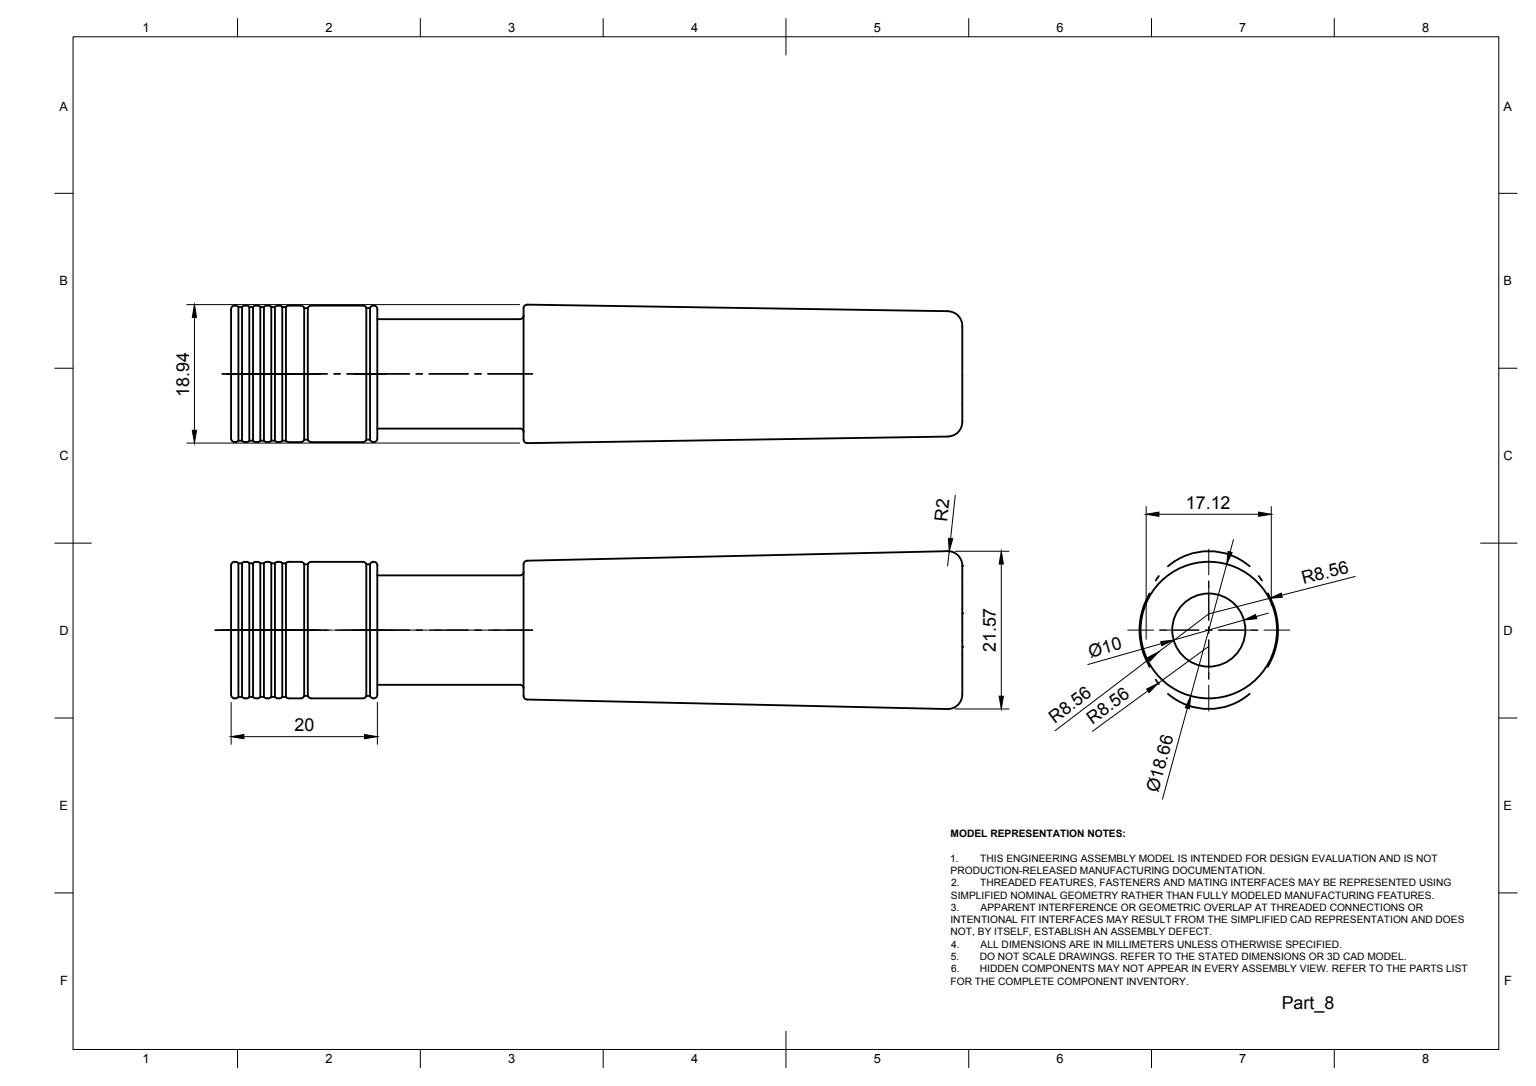
ISO-10303-21;
HEADER;
/* Generated by software containing ST-Developer
 * from STEP Tools, Inc. (www.steptools.com) 
 */

FILE_DESCRIPTION(
/* description */ ('STEP AP242 Edition 2'),
/* implementation_level */ '2;1');

FILE_NAME(
/* name */ 'Part_8.step',
/* time_stamp */ '2026-10-06T10:11:12-07:00',
/* author */ (''),
/* organization */ (''),
/* preprocessor_version */ 'ST-DEVELOPER v20.2',
/* originating_system */ 'Autodesk Translation Framework v15.15.0.0',
/* authorisation */ '');

FILE_SCHEMA (('AUTOMOTIVE_DESIGN { 1 0 10303 214 3 1 1 }'));
ENDSEC;

DATA;
#10=MECHANICAL_DESIGN_GEOMETRIC_PRESENTATION_REPRESENTATION('',(#1772,#1773,#1774,#1775,#1776,#1777,#1778,#1779,#1780,#1781,#1782,#1783,#1784),#54580);
#171=TOROIDAL_SURFACE('',#18476,0.00656151574957875,0.00199999992126171);
#172=TOROIDAL_SURFACE('',#18477,0.0065615157495791,0.00199999992126177);
#173=TOROIDAL_SURFACE('',#18479,0.0079756477610481,0.0005);
#174=TOROIDAL_SURFACE('',#18481,0.0045,0.0005);
#175=TOROIDAL_SURFACE('',#18483,0.0055,0.0005);
#176=TOROIDAL_SURFACE('',#18485,0.00882888901198444,0.0005);
#177=TOROIDAL_SURFACE('',#18487,0.00882888901198444,0.0005);
#178=TOROIDAL_SURFACE('',#18489,0.00882888901198444,0.0005);
#179=TOROIDAL_SURFACE('',#18491,0.00882888901198444,0.0005);
#180=TOROIDAL_SURFACE('',#18493,0.00882888901198444,0.0005);
#181=TOROIDAL_SURFACE('',#18495,0.00882888901198444,0.0005);
#182=TOROIDAL_SURFACE('',#18497,0.00882888901198444,0.0005);
#183=TOROIDAL_SURFACE('',#18499,0.00882888901198444,0.0005);
#184=TOROIDAL_SURFACE('',#18501,0.00882888901198444,0.0005);
#185=TOROIDAL_SURFACE('',#18503,0.00882888901198444,0.0005);
#186=TOROIDAL_SURFACE('',#18505,0.00882888901198444,0.0005);
#187=TOROIDAL_SURFACE('',#18507,0.00882888901198444,0.0005);
#188=TOROIDAL_SURFACE('',#18509,0.00882888901198444,0.0005);
#189=TOROIDAL_SURFACE('',#18511,0.00882888901198444,0.0005);
#190=TOROIDAL_SURFACE('',#18513,0.00882888901198444,0.0005);
#191=TOROIDAL_SURFACE('',#18515,0.00882888901198444,0.0005);
#323=B_SPLINE_SURFACE_WITH_KNOTS('',3,1,((#25149,#25150),(#25151,#25152),
(#25153,#25154),(#25155,#25156),(#25157,#25158),(#25159,#25160),(#25161,
#25162),(#25163,#25164),(#25165,#25166),(#25167,#25168),(#25169,#25170),
(#25171,#25172),(#25173,#25174),(#25175,#25176),(#25177,#25178),(#25179,
#25180),(#25181,#25182),(#25183,#25184),(#25185,#25186),(#25187,#25188),
(#25189,#25190),(#25191,#25192),(#25193,#25194),(#25195,#25196),(#25197,
#25198),(#25199,#25200),(#25201,#25202),(#25203,#25204),(#25205,#25206),
(#25207,#25208)),.UNSPECIFIED.,.T.,.F.,.F.,(4,1,1,1,1,1,1,1,2,1,1,1,2,1,
1,1,1,1,1,1,2,1,1,1,4),(2,2),(-1.,-0.94727121518274,-0.894542430365479,
-0.841813645548218,-0.789084860730959,-0.736356075913698,-0.683627291096437,
-0.630898506279177,-0.578169721461916,-0.558627291096437,-0.539084860730958,
-0.519542430365479,-0.5,-0.447271215182739,-0.394542430365479,-0.341813645548219,
-0.289084860730958,-0.236356075913698,-0.183627291096437,-0.130898506279177,
-0.078169721461917,-0.0586272910964371,-0.039084860730958,-0.019542430365479,
0.),(0.0270596808612465,0.997611167870436),.UNSPECIFIED.);
#324=B_SPLINE_SURFACE_WITH_KNOTS('',3,1,((#25444,#25445),(#25446,#25447),
(#25448,#25449),(#25450,#25451),(#25452,#25453),(#25454,#25455),(#25456,
#25457),(#25458,#25459),(#25460,#25461),(#25462,#25463),(#25464,#25465),
(#25466,#25467),(#25468,#25469),(#25470,#25471),(#25472,#25473),(#25474,
#25475),(#25476,#25477),(#25478,#25479),(#25480,#25481),(#25482,#25483),
(#25484,#25485),(#25486,#25487),(#25488,#25489),(#25490,#25491),(#25492,
#25493),(#25494,#25495),(#25496,#25497),(#25498,#25499),(#25500,#25501),
(#25502,#25503)),.UNSPECIFIED.,.T.,.F.,.F.,(4,1,1,1,1,1,1,1,2,1,1,1,2,1,
1,1,1,1,1,1,2,1,1,1,4),(2,2),(0.,0.0527287848172604,0.105457569634521,0.158186354451782,
0.210915139269041,0.263643924086302,0.316372708903563,0.369101493720823,
0.421830278538084,0.441372708903563,0.460915139269042,0.480457569634521,
0.5,0.552728784817261,0.605457569634521,0.658186354451781,0.710915139269042,
0.763643924086302,0.816372708903563,0.869101493720823,0.921830278538083,
0.941372708903563,0.960915139269042,0.980457569634521,1.),(0.0270596808612465,
0.997611167870436),.UNSPECIFIED.);
#343=B_SPLINE_CURVE_WITH_KNOTS('',3,(#24904,#24905,#24906,#24907,#24908,
#24909,#24910,#24911,#24912,#24913,#24914,#24915,#24916,#24917,#24918,#24919,
#24920,#24921,#24922,#24923,#24924,#24925,#24926,#24927,#24928,#24929,#24930,
#24931,#24932,#24933,#24934,#24935,#24936,#24937,#24938,#24939,#24940,#24941,
#24942,#24943,#24944,#24945,#24946,#24947,#24948,#24949,#24950,#24951,#24952,
#24953,#24954,#24955,#24956,#24957,#24958,#24959,#24960,#24961,#24962,#24963,
#24964,#24965,#24966,#24967,#24968,#24969,#24970,#24971,#24972,#24973,#24974,
#24975,#24976,#24977,#24978,#24979,#24980,#24981,#24982,#24983,#24984,#24985,
#24986,#24987,#24988,#24989,#24990,#24991,#24992,#24993,#24994,#24995,#24996,
#24997,#24998,#24999,#25000,#25001,#25002,#25003,#25004,#25005,#25006,#25007,
#25008,#25009,#25010,#25011,#25012,#25013,#25014,#25015,#25016,#25017,#25018,
#25019,#25020,#25021,#25022,#25023,#25024,#25025,#25026,#25027,#25028,#25029,
#25030,#25031,#25032,#25033,#25034,#25035,#25036,#25037,#25038,#25039,#25040,
#25041,#25042,#25043,#25044,#25045),.UNSPECIFIED.,.F.,.F.,(4,3,3,3,3,3,
3,3,3,3,3,3,3,3,3,3,3,3,3,3,3,3,3,3,3,3,3,3,3,3,3,3,3,3,3,3,3,3,3,3,3,3,
3,3,3,3,3,4),(1.65573441350565E-7,0.00176667375437257,0.00259221926243185,
0.00265001063155886,0.00353334750874515,0.00441668438593144,0.00612523623771844,
0.0070666950174903,0.00965970053988215,0.0106000425262354,0.0114833794034217,
0.0131911273471506,0.0141333900349806,0.0150167269121669,0.0167215202745876,
0.0176667375437257,0.018550074420912,0.0202567299474385,0.0212000850524709,
0.0220834219296572,0.0237972002706092,0.024733432561216,0.0265001063155886,
0.0273265094643739,0.0273834431927749,0.0282667800699612,0.0291501169471475,
0.0308585741103488,0.0318001275787063,0.0326834644558926,0.0343965954050026,
0.0353334750874515,0.0379347075752174,0.0388668225961966,0.0397501594733829,
0.0414708448549527,0.0424001701049418,0.0432835069821281,0.0450045160112871,
0.0459335176136869,0.0468168544908732,0.0485354593167441,0.0494668651224321,
0.0503502019996184,0.052066506161832,0.0530002126311772,0.0538835495083635,
0.0555994356637866),.UNSPECIFIED.);
#344=B_SPLINE_CURVE_WITH_KNOTS('',3,(#25051,#25052,#25053,#25054,#25055,
#25056,#25057,#25058,#25059,#25060,#25061,#25062,#25063,#25064,#25065,#25066,
#25067,#25068,#25069,#25070,#25071,#25072,#25073,#25074,#25075,#25076,#25077,
#25078,#25079,#25080,#25081,#25082,#25083,#25084,#25085,#25086,#25087,#25088,
#25089,#25090,#25091,#25092,#25093,#25094,#25095,#25096,#25097,#25098,#25099,
#25100,#25101,#25102,#25103,#25104,#25105,#25106,#25107,#25108,#25109,#25110,
#25111,#25112,#25113,#25114,#25115,#25116,#25117),.UNSPECIFIED.,.F.,.F.,
(4,3,3,3,3,3,3,3,3,3,3,3,3,3,3,3,3,3,3,3,3,3,4),(0.0193063570369876,0.0197413378854143,
0.0225007291837996,0.0234952979646733,0.0262508507144329,0.0272500609140882,
0.0300009722450662,0.0309993547899246,0.0337510937756994,0.0347455027219703,
0.0375012153063327,0.0385033658381765,0.041251336836966,0.0422556599874251,
0.0450014583675992,0.0460030914440076,0.0487515798982325,0.0497511536421023,
0.0525017014288658,0.053501189887995,0.0562518229594991,0.057250590934481,
0.0600019444901323),.UNSPECIFIED.);
#345=B_SPLINE_CURVE_WITH_KNOTS('',3,(#25118,#25119,#25120,#25121,#25122,
#25123,#25124,#25125,#25126,#25127,#25128,#25129,#25130,#25131,#25132,#25133,
#25134,#25135,#25136,#25137,#25138,#25139,#25140,#25141,#25142,#25143,#25144,
#25145,#25146,#25147,#25148),.UNSPECIFIED.,.F.,.F.,(4,3,3,3,3,3,3,3,3,3,
4),(0.000991839717425502,0.00375012153063327,0.00474188317058086,0.00750024306126654,
0.00848950942012792,0.0112503645918998,0.0122372989824959,0.0150004861225331,
0.0159882081557064,0.0187506076531663,0.0193063570369876),.UNSPECIFIED.);
#346=B_SPLINE_CURVE_WITH_KNOTS('',1,(#25210,#25211),.UNSPECIFIED.,.F.,.F.,
(2,2),(-0.991582441935872,-0.0329929514257554),.UNSPECIFIED.);
#347=B_SPLINE_CURVE_WITH_KNOTS('',1,(#25213,#25214),.UNSPECIFIED.,.F.,.F.,
(2,2),(-0.991765438998876,-0.0337011078849239),.UNSPECIFIED.);
#348=B_SPLINE_CURVE_WITH_KNOTS('',3,(#25216,#25217,#25218,#25219,#25220,
#25221,#25222,#25223),.UNSPECIFIED.,.F.,.F.,(4,1,1,1,1,4),(0.,0.0625,0.125,
0.15625,0.1875,0.214595707386903),.UNSPECIFIED.);
#349=B_SPLINE_CURVE_WITH_KNOTS('',3,(#25225,#25226,#25227,#25228,#25229,
#25230,#25231,#25232,#25233,#25234,#25235,#25236,#25237,#25238,#25239,#25240,
#25241,#25242,#25243),.UNSPECIFIED.,.F.,.F.,(4,3,3,3,3,3,4),(1.18815451677939E-5,
0.00305752378009468,0.257254477967242,0.499999999995986,0.742745522020828,
0.996942476194294,0.99998811883621),.UNSPECIFIED.);
#350=B_SPLINE_CURVE_WITH_KNOTS('',3,(#25245,#25246,#25247,#25248,#25249,
#25250,#25251,#25252,#25253,#25254,#25255,#25256,#25257,#25258,#25259,#25260,
#25261,#25262,#25263,#25264,#25265,#25266,#25267,#25268,#25269,#25270,#25271,
#25272,#25273,#25274,#25275,#25276,#25277,#25278,#25279),.UNSPECIFIED.,
 .F.,.F.,(4,1,1,1,1,1,1,1,1,1,1,1,1,1,1,1,1,1,1,1,1,1,1,1,1,1,1,1,1,1,1,
1,4),(0.,0.0625,0.125,0.15625,0.1875,0.21875,0.234375,0.2421875,0.25,0.2578125,
0.265625,0.28125,0.3125,0.34375,0.375,0.4375,0.5,0.5625,0.625,0.65625,0.6875,
0.71875,0.734375,0.7421875,0.75,0.7578125,0.765625,0.78125,0.8125,0.84375,
0.875,0.9375,1.),.UNSPECIFIED.);
#351=B_SPLINE_CURVE_WITH_KNOTS('',3,(#25280,#25281,#25282,#25283,#25284,
#25285,#25286,#25287,#25288,#25289,#25290,#25291,#25292,#25293,#25294,#25295),
 .UNSPECIFIED.,.F.,.F.,(4,3,3,3,3,4),(0.00305752354988625,0.25725447786239,
0.499999999961484,0.742745522020858,0.996942476194068,0.999988118836217),
 .UNSPECIFIED.);
#352=B_SPLINE_CURVE_WITH_KNOTS('',3,(#25505,#25506,#25507,#25508),
 .UNSPECIFIED.,.F.,.F.,(4,4),(1.18815450203416E-5,0.00305752354988625),
 .UNSPECIFIED.);
#353=B_SPLINE_CURVE_WITH_KNOTS('',3,(#25509,#25510,#25511,#25512,#25513,
#25514,#25515,#25516,#25517,#25518,#25519,#25520,#25521,#25522,#25523,#25524,
#25525,#25526,#25527,#25528,#25529,#25530,#25531,#25532,#25533,#25534,#25535,
#25536,#25537,#25538,#25539),.UNSPECIFIED.,.F.,.F.,(4,1,1,1,1,1,1,1,1,1,
1,1,1,1,1,1,1,1,1,1,1,1,1,1,1,1,1,1,4),(0.214595707386903,0.21875,0.234375,
0.2421875,0.25,0.2578125,0.265625,0.28125,0.3125,0.34375,0.375,0.4375,0.5,
0.5625,0.625,0.65625,0.6875,0.71875,0.734375,0.7421875,0.75,0.7578125,0.765625,
0.78125,0.8125,0.84375,0.875,0.9375,1.),.UNSPECIFIED.);
#354=B_SPLINE_CURVE_WITH_KNOTS('',3,(#25540,#25541,#25542,#25543),
 .UNSPECIFIED.,.F.,.F.,(4,4),(0.,0.000991839717425502),.UNSPECIFIED.);
#355=B_SPLINE_CURVE_WITH_KNOTS('',3,(#25546,#25547,#25548,#25549),
 .UNSPECIFIED.,.F.,.F.,(4,4),(0.,1.65573441350565E-7),.UNSPECIFIED.);
#356=B_SPLINE_CURVE_WITH_KNOTS('',3,(#25550,#25551,#25552,#25553),
 .UNSPECIFIED.,.F.,.F.,(4,4),(0.0555994356637866,0.0565335601399224),
 .UNSPECIFIED.);
#357=B_SPLINE_CURVE_WITH_KNOTS('',3,(#25562,#25563,#25564,#25565,#25566,
#25567,#25568,#25569,#25570,#25571,#25572,#25573,#25574,#25575,#25576,#25577,
#25578,#25579,#25580,#25581,#25582,#25583,#25584,#25585,#25586),
 .UNSPECIFIED.,.F.,.F.,(4,3,3,3,3,3,3,3,4),(0.,0.144356336537315,0.25,0.395552475785214,
0.5,0.64383331940147,0.75,0.898848831223356,1.),.UNSPECIFIED.);
#358=B_SPLINE_CURVE_WITH_KNOTS('',3,(#25588,#25589,#25590,#25591,#25592,
#25593,#25594,#25595,#25596,#25597,#25598,#25599,#25600,#25601,#25602,#25603,
#25604,#25605,#25606,#25607,#25608,#25609,#25610,#25611,#25612,#25613,#25614,
#25615,#25616,#25617,#25618,#25619,#25620,#25621,#25622,#25623,#25624),
 .UNSPECIFIED.,.F.,.F.,(4,3,3,3,3,3,3,3,3,3,3,3,4),(0.,0.125,0.1875,0.25,
0.3125,0.375,0.5,0.625,0.6875,0.75,0.8125,0.875,1.),.UNSPECIFIED.);
#359=B_SPLINE_CURVE_WITH_KNOTS('',3,(#25626,#25627,#25628,#25629,#25630,
#25631,#25632,#25633,#25634,#25635,#25636,#25637,#25638,#25639,#25640,#25641,
#25642,#25643,#25644,#25645,#25646,#25647,#25648,#25649,#25650),
 .UNSPECIFIED.,.F.,.F.,(4,3,3,3,3,3,3,3,4),(0.,0.144356336542805,0.25,0.395552475791052,
0.5,0.643833319408362,0.75,0.898848831228882,1.),.UNSPECIFIED.);
#360=B_SPLINE_CURVE_WITH_KNOTS('',3,(#25651,#25652,#25653,#25654,#25655,
#25656,#25657,#25658,#25659,#25660,#25661,#25662,#25663,#25664,#25665,#25666,
#25667,#25668,#25669,#25670,#25671,#25672,#25673,#25674,#25675,#25676,#25677,
#25678,#25679,#25680,#25681,#25682,#25683,#25684,#25685,#25686,#25687),
 .UNSPECIFIED.,.F.,.F.,(4,3,3,3,3,3,3,3,3,3,3,3,4),(0.,0.125,0.1875,0.25,
0.3125,0.375,0.5,0.625,0.6875,0.75,0.8125,0.875,1.),.UNSPECIFIED.);
#361=B_SPLINE_CURVE_WITH_KNOTS('',3,(#25689,#25690,#25691,#25692,#25693,
#25694,#25695,#25696,#25697,#25698,#25699,#25700,#25701),.UNSPECIFIED.,
 .F.,.F.,(4,3,3,3,4),(0.,0.393665259181331,0.5,0.894848401742748,0.999999577588646),
 .UNSPECIFIED.);
#362=B_SPLINE_CURVE_WITH_KNOTS('',3,(#25702,#25703,#25704,#25705,#25706,
#25707,#25708,#25709,#25710,#25711,#25712,#25713,#25714),.UNSPECIFIED.,
 .F.,.F.,(4,3,3,3,4),(4.22403003312878E-7,0.394848747914453,0.5,0.89366522956997,
1.),.UNSPECIFIED.);
#363=B_SPLINE_CURVE_WITH_KNOTS('',3,(#25716,#25717,#25718,#25719,#25720,
#25721,#25722,#25723,#25724,#25725,#25726,#25727,#25728),.UNSPECIFIED.,
 .F.,.F.,(4,3,3,3,4),(0.,0.39366525918135,0.5,0.894848401747474,0.999999577588569),
 .UNSPECIFIED.);
#364=B_SPLINE_CURVE_WITH_KNOTS('',3,(#25730,#25731,#25732,#25733,#25734,
#25735,#25736,#25737,#25738,#25739,#25740,#25741,#25742),.UNSPECIFIED.,
 .F.,.F.,(4,3,3,3,4),(4.22402912852314E-7,0.394848747910699,0.5,0.893665229570505,
1.),.UNSPECIFIED.);
#1512=(
BOUNDED_CURVE()
B_SPLINE_CURVE(2,(#24900,#24901,#24902),.UNSPECIFIED.,.F.,.F.)
B_SPLINE_CURVE_WITH_KNOTS((3,3),(-0.99956690722118,-2.51118997643904E-6),
 .UNSPECIFIED.)
CURVE()
GEOMETRIC_REPRESENTATION_ITEM()
RATIONAL_B_SPLINE_CURVE((0.999750853586006,0.71236441613048,0.999998554758888))
REPRESENTATION_ITEM('')
);
#1513=(
BOUNDED_CURVE()
B_SPLINE_CURVE(2,(#25047,#25048,#25049),.UNSPECIFIED.,.F.,.F.)
B_SPLINE_CURVE_WITH_KNOTS((3,3),(-0.999613386882244,0.),.UNSPECIFIED.)
CURVE()
GEOMETRIC_REPRESENTATION_ITEM()
RATIONAL_B_SPLINE_CURVE((0.999776843008427,0.711394956192752,1.))
REPRESENTATION_ITEM('')
);
#1530=(
BOUNDED_SURFACE()
B_SPLINE_SURFACE(3,2,((#24841,#24842,#24843),(#24844,#24845,#24846),(#24847,
#24848,#24849),(#24850,#24851,#24852),(#24853,#24854,#24855),(#24856,#24857,
#24858),(#24859,#24860,#24861),(#24862,#24863,#24864),(#24865,#24866,#24867),
(#24868,#24869,#24870),(#24871,#24872,#24873),(#24874,#24875,#24876),(#24877,
#24878,#24879),(#24880,#24881,#24882),(#24883,#24884,#24885),(#24886,#24887,
#24888),(#24889,#24890,#24891),(#24892,#24893,#24894),(#24895,#24896,#24897)),
 .UNSPECIFIED.,.T.,.F.,.F.)
B_SPLINE_SURFACE_WITH_KNOTS((4,1,1,1,1,1,1,1,1,1,1,1,1,1,1,1,4),(3,3),(-0.056131150341711,
-0.0526229534453541,-0.0491147565489971,-0.0456065596526402,-0.0420983627562833,
-0.0385901658599263,-0.0350819689635694,-0.0315737720672124,-0.0280655751708555,
-0.0245573782744986,-0.0210491813781416,-0.0175409844817847,-0.0140327875854278,
-0.0105245906890708,-0.0070163937927139,-0.003508196896357,0.),(0.,1.),
 .UNSPECIFIED.)
GEOMETRIC_REPRESENTATION_ITEM()
RATIONAL_B_SPLINE_SURFACE(((1.,0.712239066951905,1.),(1.,0.711110760308393,
1.),(1.,0.708331161318748,1.),(1.,0.701023190412799,1.),(1.,0.701644224301599,
1.),(1.,0.70884038203116,1.),(1.,0.712835506198471,1.),(1.,0.715218629500482,
1.),(1.,0.715102433806893,1.),(1.,0.712501311419114,1.),(1.,0.708334487423287,
1.),(1.,0.701010241546403,1.),(1.,0.701662301810715,1.),(1.,0.708859933389416,
1.),(1.,0.712846256318991,1.),(1.,0.715219419684522,1.),(1.,0.715101001179818,
1.),(1.,0.713367373595416,1.),(1.,0.712239066951905,1.)))
REPRESENTATION_ITEM('')
SURFACE()
);
#1531=(
BOUNDED_SURFACE()
B_SPLINE_SURFACE(3,2,((#25782,#25783,#25784),(#25785,#25786,#25787),(#25788,
#25789,#25790),(#25791,#25792,#25793),(#25794,#25795,#25796),(#25797,#25798,
#25799),(#25800,#25801,#25802),(#25803,#25804,#25805),(#25806,#25807,#25808),
(#25809,#25810,#25811),(#25812,#25813,#25814),(#25815,#25816,#25817),(#25818,
#25819,#25820),(#25821,#25822,#25823),(#25824,#25825,#25826),(#25827,#25828,
#25829),(#25830,#25831,#25832),(#25833,#25834,#25835),(#25836,#25837,#25838)),
 .UNSPECIFIED.,.T.,.F.,.F.)
B_SPLINE_SURFACE_WITH_KNOTS((4,1,1,1,1,1,1,1,1,1,1,1,1,1,1,1,4),(3,3),(0.056131150341711,
0.0596393472380679,0.0631475441344249,0.0666557410307818,0.0701639379271387,
0.0736721348234957,0.0771803317198526,0.0806885286162096,0.0841967255125665,
0.0877049224089234,0.0912131193052804,0.0947213162016373,0.0982295130979942,
0.101737709994351,0.105245906890708,0.108754103787065,0.112262300683422),
(0.,1.),.UNSPECIFIED.)
GEOMETRIC_REPRESENTATION_ITEM()
RATIONAL_B_SPLINE_SURFACE(((1.,0.712239066951905,1.),(1.,0.711110760308393,
1.),(1.,0.708331161318748,1.),(1.,0.701023190412799,1.),(1.,0.701644224301599,
1.),(1.,0.70884038203116,1.),(1.,0.712835506198471,1.),(1.,0.715218629500482,
1.),(1.,0.715102433806893,1.),(1.,0.712501311419114,1.),(1.,0.708334487423287,
1.),(1.,0.701010241546403,1.),(1.,0.701662301810715,1.),(1.,0.708859933389416,
1.),(1.,0.712846256318991,1.),(1.,0.715219419684522,1.),(1.,0.715101001179818,
1.),(1.,0.713367373595416,1.),(1.,0.712239066951905,1.)))
REPRESENTATION_ITEM('')
SURFACE()
);
#1744=SHAPE_REPRESENTATION_RELATIONSHIP('SRR','None',#54631,#1758);
#1758=ADVANCED_BREP_SHAPE_REPRESENTATION('',(#1802),#54567);
#1772=STYLED_ITEM('',(#54712),#16847);
#1773=STYLED_ITEM('',(#54712),#16848);
#1774=STYLED_ITEM('',(#54711),#16850);
#1775=STYLED_ITEM('',(#54712),#16868);
#1776=STYLED_ITEM('',(#54712),#16869);
#1777=STYLED_ITEM('',(#54712),#16871);
#1778=STYLED_ITEM('',(#54712),#16872);
#1779=STYLED_ITEM('',(#54712),#16873);
#1780=STYLED_ITEM('',(#54712),#16874);
#1781=STYLED_ITEM('',(#54712),#16875);
#1782=STYLED_ITEM('',(#54712),#16876);
#1783=STYLED_ITEM('',(#54712),#16895);
#1784=STYLED_ITEM('',(#54710),#1802);
#1802=MANIFOLD_SOLID_BREP('Body1',#17667);
#2000=LINE('',#25302,#2593);
#2001=LINE('',#25310,#2594);
#2002=LINE('',#25320,#2595);
#2003=LINE('',#25328,#2596);
#2004=LINE('',#25346,#2597);
#2005=LINE('',#25354,#2598);
#2006=LINE('',#25360,#2599);
#2007=LINE('',#25368,#2600);
#2008=LINE('',#25378,#2601);
#2009=LINE('',#25386,#2602);
#2010=LINE('',#25392,#2603);
#2011=LINE('',#25402,#2604);
#2012=LINE('',#25408,#2605);
#2013=LINE('',#25418,#2606);
#2014=LINE('',#25424,#2607);
#2015=LINE('',#25434,#2608);
#2016=LINE('',#25440,#2609);
#2593=VECTOR('',#20912,0.005);
#2594=VECTOR('',#20921,0.0074756477610481);
#2595=VECTOR('',#20932,0.00932888901198444);
#2596=VECTOR('',#20941,0.00932888901198444);
#2597=VECTOR('',#20962,0.00898940279602035);
#2598=VECTOR('',#20971,0.00912888901198444);
#2599=VECTOR('',#20978,0.00932888901198444);
#2600=VECTOR('',#20987,0.00932888901198444);
#2601=VECTOR('',#20998,0.00898940279602035);
#2602=VECTOR('',#21007,0.00912888901198443);
#2603=VECTOR('',#21014,0.00932888901198444);
#2604=VECTOR('',#21025,0.0091288890119844);
#2605=VECTOR('',#21032,0.00932888901198444);
#2606=VECTOR('',#21043,0.00912888901198441);
#2607=VECTOR('',#21050,0.00932888901198444);
#2608=VECTOR('',#21061,0.00912888901198442);
#2609=VECTOR('',#21068,0.00932888901198444);
#3186=CYLINDRICAL_SURFACE('',#18395,0.005);
#3187=CYLINDRICAL_SURFACE('',#18400,0.0074756477610481);
#3188=CYLINDRICAL_SURFACE('',#18404,0.00932888901198444);
#3189=CYLINDRICAL_SURFACE('',#18409,0.00932888901198444);
#3190=CYLINDRICAL_SURFACE('',#18418,0.00898940279602035);
#3191=CYLINDRICAL_SURFACE('',#18422,0.00912888901198444);
#3192=CYLINDRICAL_SURFACE('',#18426,0.00932888901198444);
#3193=CYLINDRICAL_SURFACE('',#18430,0.00932888901198444);
#3194=CYLINDRICAL_SURFACE('',#18434,0.00898940279602035);
#3195=CYLINDRICAL_SURFACE('',#18438,0.00912888901198443);
#3196=CYLINDRICAL_SURFACE('',#18442,0.00932888901198444);
#3197=CYLINDRICAL_SURFACE('',#18446,0.0091288890119844);
#3198=CYLINDRICAL_SURFACE('',#18450,0.00932888901198444);
#3199=CYLINDRICAL_SURFACE('',#18454,0.00912888901198441);
#3200=CYLINDRICAL_SURFACE('',#18458,0.00932888901198444);
#3201=CYLINDRICAL_SURFACE('',#18462,0.00912888901198442);
#3202=CYLINDRICAL_SURFACE('',#18466,0.00932888901198444);
#3203=CYLINDRICAL_SURFACE('',#18475,0.0019998995087818);
#3204=CYLINDRICAL_SURFACE('',#18478,0.00199989950878194);
#3479=FACE_BOUND('',#4746,.T.);
#3480=FACE_BOUND('',#4748,.T.);
#3481=FACE_BOUND('',#4764,.T.);
#3731=FACE_OUTER_BOUND('',#4739,.T.);
#3732=FACE_OUTER_BOUND('',#4740,.T.);
#3733=FACE_OUTER_BOUND('',#4741,.T.);
#3734=FACE_OUTER_BOUND('',#4742,.T.);
#3735=FACE_OUTER_BOUND('',#4743,.T.);
#3736=FACE_OUTER_BOUND('',#4744,.T.);
#3737=FACE_OUTER_BOUND('',#4745,.T.);
#3738=FACE_OUTER_BOUND('',#4747,.T.);
#3739=FACE_OUTER_BOUND('',#4749,.T.);
#3740=FACE_OUTER_BOUND('',#4750,.T.);
#3741=FACE_OUTER_BOUND('',#4751,.T.);
#3742=FACE_OUTER_BOUND('',#4752,.T.);
#3743=FACE_OUTER_BOUND('',#4753,.T.);
#3744=FACE_OUTER_BOUND('',#4754,.T.);
#3745=FACE_OUTER_BOUND('',#4755,.T.);
#3746=FACE_OUTER_BOUND('',#4756,.T.);
#3747=FACE_OUTER_BOUND('',#4757,.T.);
#3748=FACE_OUTER_BOUND('',#4758,.T.);
#3749=FACE_OUTER_BOUND('',#4759,.T.);
#3750=FACE_OUTER_BOUND('',#4760,.T.);
#3751=FACE_OUTER_BOUND('',#4761,.T.);
#3752=FACE_OUTER_BOUND('',#4762,.T.);
#3753=FACE_OUTER_BOUND('',#4763,.T.);
#3754=FACE_OUTER_BOUND('',#4765,.T.);
#3755=FACE_OUTER_BOUND('',#4766,.T.);
#3756=FACE_OUTER_BOUND('',#4767,.T.);
#3757=FACE_OUTER_BOUND('',#4768,.T.);
#3758=FACE_OUTER_BOUND('',#4769,.T.);
#3759=FACE_OUTER_BOUND('',#4770,.T.);
#3760=FACE_OUTER_BOUND('',#4771,.T.);
#3761=FACE_OUTER_BOUND('',#4772,.T.);
#3762=FACE_OUTER_BOUND('',#4773,.T.);
#3763=FACE_OUTER_BOUND('',#4774,.T.);
#3764=FACE_OUTER_BOUND('',#4775,.T.);
#3765=FACE_OUTER_BOUND('',#4776,.T.);
#3766=FACE_OUTER_BOUND('',#4777,.T.);
#3767=FACE_OUTER_BOUND('',#4778,.T.);
#3768=FACE_OUTER_BOUND('',#4779,.T.);
#3769=FACE_OUTER_BOUND('',#4780,.T.);
#3770=FACE_OUTER_BOUND('',#4781,.T.);
#3771=FACE_OUTER_BOUND('',#4782,.T.);
#3772=FACE_OUTER_BOUND('',#4783,.T.);
#3773=FACE_OUTER_BOUND('',#4784,.T.);
#3774=FACE_OUTER_BOUND('',#4785,.T.);
#3775=FACE_OUTER_BOUND('',#4786,.T.);
#3776=FACE_OUTER_BOUND('',#4787,.T.);
#3777=FACE_OUTER_BOUND('',#4788,.T.);
#3778=FACE_OUTER_BOUND('',#4789,.T.);
#3779=FACE_OUTER_BOUND('',#4790,.T.);
#4739=EDGE_LOOP('',(#12179,#12180,#12181,#12182,#12183));
#4740=EDGE_LOOP('',(#12184,#12185,#12186,#12187,#12188,#12189,#12190));
#4741=EDGE_LOOP('',(#12191,#12192,#12193,#12194,#12195,#12196));
#4742=EDGE_LOOP('',(#12197,#12198,#12199,#12200,#12201));
#4743=EDGE_LOOP('',(#12202,#12203,#12204,#12205,#12206,#12207));
#4744=EDGE_LOOP('',(#12208,#12209,#12210,#12211,#12212));
#4745=EDGE_LOOP('',(#12213));
#4746=EDGE_LOOP('',(#12214));
#4747=EDGE_LOOP('',(#12215));
#4748=EDGE_LOOP('',(#12216));
#4749=EDGE_LOOP('',(#12217,#12218,#12219,#12220,#12221));
#4750=EDGE_LOOP('',(#12222,#12223,#12224,#12225,#12226));
#4751=EDGE_LOOP('',(#12227,#12228,#12229,#12230,#12231));
#4752=EDGE_LOOP('',(#12232,#12233,#12234,#12235,#12236));
#4753=EDGE_LOOP('',(#12237,#12238,#12239,#12240,#12241));
#4754=EDGE_LOOP('',(#12242,#12243,#12244,#12245,#12246));
#4755=EDGE_LOOP('',(#12247,#12248,#12249,#12250,#12251));
#4756=EDGE_LOOP('',(#12252,#12253,#12254,#12255,#12256));
#4757=EDGE_LOOP('',(#12257,#12258,#12259,#12260,#12261));
#4758=EDGE_LOOP('',(#12262,#12263,#12264,#12265,#12266));
#4759=EDGE_LOOP('',(#12267,#12268,#12269,#12270,#12271));
#4760=EDGE_LOOP('',(#12272,#12273,#12274,#12275,#12276));
#4761=EDGE_LOOP('',(#12277,#12278,#12279,#12280,#12281));
#4762=EDGE_LOOP('',(#12282,#12283,#12284,#12285,#12286,#12287));
#4763=EDGE_LOOP('',(#12288,#12289,#12290));
#4764=EDGE_LOOP('',(#12291));
#4765=EDGE_LOOP('',(#12292));
#4766=EDGE_LOOP('',(#12293,#12294,#12295,#12296));
#4767=EDGE_LOOP('',(#12297,#12298,#12299,#12300));
#4768=EDGE_LOOP('',(#12301,#12302,#12303,#12304,#12305));
#4769=EDGE_LOOP('',(#12306,#12307,#12308,#12309));
#4770=EDGE_LOOP('',(#12310,#12311,#12312,#12313,#12314));
#4771=EDGE_LOOP('',(#12315,#12316,#12317,#12318,#12319));
#4772=EDGE_LOOP('',(#12320,#12321,#12322,#12323,#12324));
#4773=EDGE_LOOP('',(#12325,#12326,#12327,#12328,#12329));
#4774=EDGE_LOOP('',(#12330,#12331,#12332,#12333,#12334));
#4775=EDGE_LOOP('',(#12335,#12336,#12337,#12338,#12339,#12340));
#4776=EDGE_LOOP('',(#12341,#12342,#12343,#12344,#12345,#12346));
#4777=EDGE_LOOP('',(#12347,#12348,#12349,#12350));
#4778=EDGE_LOOP('',(#12351,#12352,#12353,#12354,#12355,#12356));
#4779=EDGE_LOOP('',(#12357,#12358,#12359,#12360));
#4780=EDGE_LOOP('',(#12361,#12362,#12363,#12364,#12365,#12366));
#4781=EDGE_LOOP('',(#12367,#12368,#12369,#12370));
#4782=EDGE_LOOP('',(#12371,#12372,#12373,#12374));
#4783=EDGE_LOOP('',(#12375,#12376,#12377,#12378,#12379,#12380));
#4784=EDGE_LOOP('',(#12381,#12382,#12383,#12384));
#4785=EDGE_LOOP('',(#12385,#12386,#12387,#12388,#12389,#12390));
#4786=EDGE_LOOP('',(#12391,#12392,#12393,#12394,#12395));
#4787=EDGE_LOOP('',(#12396,#12397,#12398,#12399));
#4788=EDGE_LOOP('',(#12400,#12401,#12402,#12403,#12404,#12405));
#4789=EDGE_LOOP('',(#12406,#12407,#12408,#12409));
#4790=EDGE_LOOP('',(#12410,#12411,#12412,#12413,#12414));
#5993=CIRCLE('',#18396,0.005);
#5994=CIRCLE('',#18397,0.005);
#5995=CIRCLE('',#18398,0.005);
#5996=CIRCLE('',#18399,0.005);
#5997=CIRCLE('',#18401,0.0074756477610481);
#5998=CIRCLE('',#18402,0.0074756477610481);
#5999=CIRCLE('',#18403,0.0074756477610481);
#6000=CIRCLE('',#18405,0.00932888901198444);
#6001=CIRCLE('',#18406,0.00932888901198444);
#6002=CIRCLE('',#18407,0.00932888901198444);
#6003=CIRCLE('',#18408,0.00932888901198444);
#6004=CIRCLE('',#18410,0.00932888901198444);
#6005=CIRCLE('',#18411,0.00932888901198444);
#6006=CIRCLE('',#18412,0.00932888901198444);
#6007=CIRCLE('',#18414,0.00882888901198444);
#6008=CIRCLE('',#18415,0.0055);
#6009=CIRCLE('',#18417,0.00882888901198444);
#6010=CIRCLE('',#18419,0.00898940279602035);
#6011=CIRCLE('',#18420,0.00898940279602035);
#6012=CIRCLE('',#18421,0.00898940279602035);
#6013=CIRCLE('',#18423,0.00912888901198444);
#6014=CIRCLE('',#18424,0.00912888901198444);
#6015=CIRCLE('',#18425,0.00912888901198444);
#6016=CIRCLE('',#18427,0.00932888901198444);
#6017=CIRCLE('',#18428,0.00932888901198444);
#6018=CIRCLE('',#18429,0.00932888901198444);
#6019=CIRCLE('',#18431,0.00932888901198444);
#6020=CIRCLE('',#18432,0.00932888901198444);
#6021=CIRCLE('',#18433,0.00932888901198444);
#6022=CIRCLE('',#18435,0.00898940279602035);
#6023=CIRCLE('',#18436,0.00898940279602035);
#6024=CIRCLE('',#18437,0.00898940279602035);
#6025=CIRCLE('',#18439,0.00912888901198443);
#6026=CIRCLE('',#18440,0.00912888901198443);
#6027=CIRCLE('',#18441,0.00912888901198443);
#6028=CIRCLE('',#18443,0.00932888901198444);
#6029=CIRCLE('',#18444,0.00932888901198444);
#6030=CIRCLE('',#18445,0.00932888901198444);
#6031=CIRCLE('',#18447,0.0091288890119844);
#6032=CIRCLE('',#18448,0.0091288890119844);
#6033=CIRCLE('',#18449,0.0091288890119844);
#6034=CIRCLE('',#18451,0.00932888901198444);
#6035=CIRCLE('',#18452,0.00932888901198444);
#6036=CIRCLE('',#18453,0.00932888901198444);
#6037=CIRCLE('',#18455,0.00912888901198441);
#6038=CIRCLE('',#18456,0.00912888901198441);
#6039=CIRCLE('',#18457,0.00912888901198441);
#6040=CIRCLE('',#18459,0.00932888901198444);
#6041=CIRCLE('',#18460,0.00932888901198444);
#6042=CIRCLE('',#18461,0.00932888901198444);
#6043=CIRCLE('',#18463,0.00912888901198442);
#6044=CIRCLE('',#18464,0.00912888901198442);
#6045=CIRCLE('',#18465,0.00912888901198442);
#6046=CIRCLE('',#18467,0.00932888901198444);
#6047=CIRCLE('',#18468,0.00932888901198444);
#6048=CIRCLE('',#18469,0.00932888901198444);
#6049=CIRCLE('',#18471,0.0079756477610481);
#6050=CIRCLE('',#18473,0.0045);
#6051=CIRCLE('',#18480,0.0005);
#6052=CIRCLE('',#18482,0.0005);
#6053=CIRCLE('',#18484,0.0005);
#6054=CIRCLE('',#18486,0.0005);
#6055=CIRCLE('',#18488,0.0005);
#6056=CIRCLE('',#18490,0.0005);
#6057=CIRCLE('',#18492,0.0005);
#6058=CIRCLE('',#18494,0.0005);
#6059=CIRCLE('',#18496,0.0005);
#6060=CIRCLE('',#18498,0.0005);
#6061=CIRCLE('',#18500,0.0005);
#6062=CIRCLE('',#18502,0.0005);
#6063=CIRCLE('',#18504,0.0005);
#6064=CIRCLE('',#18506,0.0005);
#6065=CIRCLE('',#18508,0.0005);
#6066=CIRCLE('',#18510,0.0005);
#6067=CIRCLE('',#18512,0.0005);
#6068=CIRCLE('',#18514,0.0005);
#6069=CIRCLE('',#18516,0.0005);
#6896=VERTEX_POINT('',#24898);
#6897=VERTEX_POINT('',#24899);
#6898=VERTEX_POINT('',#24903);
#6899=VERTEX_POINT('',#25046);
#6900=VERTEX_POINT('',#25050);
#6901=VERTEX_POINT('',#25209);
#6902=VERTEX_POINT('',#25212);
#6903=VERTEX_POINT('',#25215);
#6904=VERTEX_POINT('',#25224);
#6905=VERTEX_POINT('',#25244);
#6906=VERTEX_POINT('',#25297);
#6907=VERTEX_POINT('',#25298);
#6908=VERTEX_POINT('',#25301);
#6909=VERTEX_POINT('',#25303);
#6910=VERTEX_POINT('',#25307);
#6911=VERTEX_POINT('',#25309);
#6912=VERTEX_POINT('',#25311);
#6913=VERTEX_POINT('',#25315);
#6914=VERTEX_POINT('',#25316);
#6915=VERTEX_POINT('',#25319);
#6916=VERTEX_POINT('',#25321);
#6917=VERTEX_POINT('',#25325);
#6918=VERTEX_POINT('',#25327);
#6919=VERTEX_POINT('',#25329);
#6920=VERTEX_POINT('',#25333);
#6921=VERTEX_POINT('',#25335);
#6922=VERTEX_POINT('',#25338);
#6923=VERTEX_POINT('',#25341);
#6924=VERTEX_POINT('',#25342);
#6925=VERTEX_POINT('',#25345);
#6926=VERTEX_POINT('',#25349);
#6927=VERTEX_POINT('',#25350);
#6928=VERTEX_POINT('',#25353);
#6929=VERTEX_POINT('',#25357);
#6930=VERTEX_POINT('',#25359);
#6931=VERTEX_POINT('',#25361);
#6932=VERTEX_POINT('',#25365);
#6933=VERTEX_POINT('',#25367);
#6934=VERTEX_POINT('',#25369);
#6935=VERTEX_POINT('',#25373);
#6936=VERTEX_POINT('',#25374);
#6937=VERTEX_POINT('',#25377);
#6938=VERTEX_POINT('',#25381);
#6939=VERTEX_POINT('',#25382);
#6940=VERTEX_POINT('',#25385);
#6941=VERTEX_POINT('',#25389);
#6942=VERTEX_POINT('',#25391);
#6943=VERTEX_POINT('',#25393);
#6944=VERTEX_POINT('',#25397);
#6945=VERTEX_POINT('',#25398);
#6946=VERTEX_POINT('',#25401);
#6947=VERTEX_POINT('',#25405);
#6948=VERTEX_POINT('',#25407);
#6949=VERTEX_POINT('',#25409);
#6950=VERTEX_POINT('',#25413);
#6951=VERTEX_POINT('',#25414);
#6952=VERTEX_POINT('',#25417);
#6953=VERTEX_POINT('',#25421);
#6954=VERTEX_POINT('',#25423);
#6955=VERTEX_POINT('',#25425);
#6956=VERTEX_POINT('',#25429);
#6957=VERTEX_POINT('',#25430);
#6958=VERTEX_POINT('',#25433);
#6959=VERTEX_POINT('',#25437);
#6960=VERTEX_POINT('',#25439);
#6961=VERTEX_POINT('',#25441);
#6962=VERTEX_POINT('',#25504);
#6963=VERTEX_POINT('',#25545);
#6964=VERTEX_POINT('',#25554);
#6965=VERTEX_POINT('',#25557);
#6966=VERTEX_POINT('',#25560);
#6967=VERTEX_POINT('',#25561);
#6968=VERTEX_POINT('',#25587);
#6969=VERTEX_POINT('',#25625);
#8881=EDGE_CURVE('',#6896,#6897,#1512,.T.);
#8882=EDGE_CURVE('',#6898,#6896,#343,.T.);
#8883=EDGE_CURVE('',#6898,#6899,#1513,.T.);
#8884=EDGE_CURVE('',#6900,#6899,#344,.T.);
#8885=EDGE_CURVE('',#6897,#6900,#345,.T.);
#8886=EDGE_CURVE('',#6900,#6901,#346,.T.);
#8887=EDGE_CURVE('',#6899,#6902,#347,.T.);
#8888=EDGE_CURVE('',#6902,#6903,#348,.F.);
#8889=EDGE_CURVE('',#6903,#6904,#349,.F.);
#8890=EDGE_CURVE('',#6904,#6905,#350,.F.);
#8891=EDGE_CURVE('',#6905,#6901,#351,.F.);
#8892=EDGE_CURVE('',#6906,#6907,#5993,.T.);
#8893=EDGE_CURVE('',#6907,#6906,#5994,.T.);
#8894=EDGE_CURVE('',#6906,#6908,#2000,.T.);
#8895=EDGE_CURVE('',#6908,#6909,#5995,.F.);
#8896=EDGE_CURVE('',#6909,#6908,#5996,.F.);
#8897=EDGE_CURVE('',#6910,#6910,#5997,.T.);
#8898=EDGE_CURVE('',#6910,#6911,#2001,.T.);
#8899=EDGE_CURVE('',#6911,#6912,#5998,.F.);
#8900=EDGE_CURVE('',#6912,#6911,#5999,.F.);
#8901=EDGE_CURVE('',#6913,#6914,#6000,.T.);
#8902=EDGE_CURVE('',#6914,#6913,#6001,.T.);
#8903=EDGE_CURVE('',#6913,#6915,#2002,.T.);
#8904=EDGE_CURVE('',#6915,#6916,#6002,.F.);
#8905=EDGE_CURVE('',#6916,#6915,#6003,.F.);
#8906=EDGE_CURVE('',#6917,#6917,#6004,.F.);
#8907=EDGE_CURVE('',#6917,#6918,#2003,.T.);
#8908=EDGE_CURVE('',#6918,#6919,#6005,.F.);
#8909=EDGE_CURVE('',#6919,#6918,#6006,.F.);
#8910=EDGE_CURVE('',#6920,#6920,#6007,.F.);
#8911=EDGE_CURVE('',#6921,#6921,#6008,.T.);
#8912=EDGE_CURVE('',#6922,#6922,#6009,.T.);
#8913=EDGE_CURVE('',#6923,#6924,#6010,.T.);
#8914=EDGE_CURVE('',#6924,#6923,#6011,.T.);
#8915=EDGE_CURVE('',#6924,#6925,#2004,.T.);
#8916=EDGE_CURVE('',#6925,#6925,#6012,.T.);
#8917=EDGE_CURVE('',#6926,#6927,#6013,.T.);
#8918=EDGE_CURVE('',#6927,#6926,#6014,.T.);
#8919=EDGE_CURVE('',#6927,#6928,#2005,.T.);
#8920=EDGE_CURVE('',#6928,#6928,#6015,.T.);
#8921=EDGE_CURVE('',#6929,#6929,#6016,.F.);
#8922=EDGE_CURVE('',#6929,#6930,#2006,.T.);
#8923=EDGE_CURVE('',#6930,#6931,#6017,.F.);
#8924=EDGE_CURVE('',#6931,#6930,#6018,.F.);
#8925=EDGE_CURVE('',#6932,#6932,#6019,.F.);
#8926=EDGE_CURVE('',#6932,#6933,#2007,.T.);
#8927=EDGE_CURVE('',#6933,#6934,#6020,.F.);
#8928=EDGE_CURVE('',#6934,#6933,#6021,.F.);
#8929=EDGE_CURVE('',#6935,#6936,#6022,.T.);
#8930=EDGE_CURVE('',#6936,#6935,#6023,.T.);
#8931=EDGE_CURVE('',#6936,#6937,#2008,.T.);
#8932=EDGE_CURVE('',#6937,#6937,#6024,.T.);
#8933=EDGE_CURVE('',#6938,#6939,#6025,.T.);
#8934=EDGE_CURVE('',#6939,#6938,#6026,.T.);
#8935=EDGE_CURVE('',#6939,#6940,#2009,.T.);
#8936=EDGE_CURVE('',#6940,#6940,#6027,.T.);
#8937=EDGE_CURVE('',#6941,#6941,#6028,.F.);
#8938=EDGE_CURVE('',#6941,#6942,#2010,.T.);
#8939=EDGE_CURVE('',#6942,#6943,#6029,.F.);
#8940=EDGE_CURVE('',#6943,#6942,#6030,.F.);
#8941=EDGE_CURVE('',#6944,#6945,#6031,.T.);
#8942=EDGE_CURVE('',#6945,#6944,#6032,.T.);
#8943=EDGE_CURVE('',#6945,#6946,#2011,.T.);
#8944=EDGE_CURVE('',#6946,#6946,#6033,.T.);
#8945=EDGE_CURVE('',#6947,#6947,#6034,.F.);
#8946=EDGE_CURVE('',#6947,#6948,#2012,.T.);
#8947=EDGE_CURVE('',#6948,#6949,#6035,.F.);
#8948=EDGE_CURVE('',#6949,#6948,#6036,.F.);
#8949=EDGE_CURVE('',#6950,#6951,#6037,.T.);
#8950=EDGE_CURVE('',#6951,#6950,#6038,.T.);
#8951=EDGE_CURVE('',#6951,#6952,#2013,.T.);
#8952=EDGE_CURVE('',#6952,#6952,#6039,.T.);
#8953=EDGE_CURVE('',#6953,#6953,#6040,.F.);
#8954=EDGE_CURVE('',#6953,#6954,#2014,.T.);
#8955=EDGE_CURVE('',#6954,#6955,#6041,.F.);
#8956=EDGE_CURVE('',#6955,#6954,#6042,.F.);
#8957=EDGE_CURVE('',#6956,#6957,#6043,.T.);
#8958=EDGE_CURVE('',#6957,#6956,#6044,.T.);
#8959=EDGE_CURVE('',#6957,#6958,#2015,.T.);
#8960=EDGE_CURVE('',#6958,#6958,#6045,.T.);
#8961=EDGE_CURVE('',#6959,#6959,#6046,.F.);
#8962=EDGE_CURVE('',#6959,#6960,#2016,.T.);
#8963=EDGE_CURVE('',#6960,#6961,#6047,.F.);
#8964=EDGE_CURVE('',#6961,#6960,#6048,.F.);
#8965=EDGE_CURVE('',#6901,#6962,#352,.F.);
#8966=EDGE_CURVE('',#6962,#6902,#353,.F.);
#8967=EDGE_CURVE('',#6899,#6897,#354,.T.);
#8968=EDGE_CURVE('',#6963,#6898,#355,.T.);
#8969=EDGE_CURVE('',#6896,#6963,#356,.T.);
#8970=EDGE_CURVE('',#6964,#6964,#6049,.T.);
#8971=EDGE_CURVE('',#6965,#6965,#6050,.F.);
#8972=EDGE_CURVE('',#6966,#6967,#357,.T.);
#8973=EDGE_CURVE('',#6967,#6968,#358,.T.);
#8974=EDGE_CURVE('',#6968,#6969,#359,.T.);
#8975=EDGE_CURVE('',#6969,#6966,#360,.T.);
#8976=EDGE_CURVE('',#6904,#6969,#361,.F.);
#8977=EDGE_CURVE('',#6966,#6903,#362,.F.);
#8978=EDGE_CURVE('',#6967,#6962,#363,.T.);
#8979=EDGE_CURVE('',#6905,#6968,#364,.T.);
#8980=EDGE_CURVE('',#6964,#6912,#6051,.T.);
#8981=EDGE_CURVE('',#6907,#6965,#6052,.T.);
#8982=EDGE_CURVE('',#6921,#6909,#6053,.T.);
#8983=EDGE_CURVE('',#6914,#6920,#6054,.T.);
#8984=EDGE_CURVE('',#6926,#6916,#6055,.T.);
#8985=EDGE_CURVE('',#6938,#6934,#6056,.T.);
#8986=EDGE_CURVE('',#6928,#6932,#6057,.T.);
#8987=EDGE_CURVE('',#6956,#6961,#6058,.T.);
#8988=EDGE_CURVE('',#6940,#6959,#6059,.T.);
#8989=EDGE_CURVE('',#6950,#6955,#6060,.T.);
#8990=EDGE_CURVE('',#6958,#6953,#6061,.T.);
#8991=EDGE_CURVE('',#6952,#6947,#6062,.T.);
#8992=EDGE_CURVE('',#6944,#6949,#6063,.T.);
#8993=EDGE_CURVE('',#6946,#6941,#6064,.T.);
#8994=EDGE_CURVE('',#6935,#6943,#6065,.T.);
#8995=EDGE_CURVE('',#6922,#6919,#6066,.T.);
#8996=EDGE_CURVE('',#6925,#6917,#6067,.T.);
#8997=EDGE_CURVE('',#6923,#6931,#6068,.T.);
#8998=EDGE_CURVE('',#6937,#6929,#6069,.T.);
#12179=ORIENTED_EDGE('',*,*,#8881,.F.);
#12180=ORIENTED_EDGE('',*,*,#8882,.F.);
#12181=ORIENTED_EDGE('',*,*,#8883,.T.);
#12182=ORIENTED_EDGE('',*,*,#8884,.F.);
#12183=ORIENTED_EDGE('',*,*,#8885,.F.);
#12184=ORIENTED_EDGE('',*,*,#8886,.F.);
#12185=ORIENTED_EDGE('',*,*,#8884,.T.);
#12186=ORIENTED_EDGE('',*,*,#8887,.T.);
#12187=ORIENTED_EDGE('',*,*,#8888,.T.);
#12188=ORIENTED_EDGE('',*,*,#8889,.T.);
#12189=ORIENTED_EDGE('',*,*,#8890,.T.);
#12190=ORIENTED_EDGE('',*,*,#8891,.T.);
#12191=ORIENTED_EDGE('',*,*,#8892,.T.);
#12192=ORIENTED_EDGE('',*,*,#8893,.T.);
#12193=ORIENTED_EDGE('',*,*,#8894,.T.);
#12194=ORIENTED_EDGE('',*,*,#8895,.T.);
#12195=ORIENTED_EDGE('',*,*,#8896,.T.);
#12196=ORIENTED_EDGE('',*,*,#8894,.F.);
#12197=ORIENTED_EDGE('',*,*,#8897,.T.);
#12198=ORIENTED_EDGE('',*,*,#8898,.T.);
#12199=ORIENTED_EDGE('',*,*,#8899,.T.);
#12200=ORIENTED_EDGE('',*,*,#8900,.T.);
#12201=ORIENTED_EDGE('',*,*,#8898,.F.);
#12202=ORIENTED_EDGE('',*,*,#8901,.T.);
#12203=ORIENTED_EDGE('',*,*,#8902,.T.);
#12204=ORIENTED_EDGE('',*,*,#8903,.T.);
#12205=ORIENTED_EDGE('',*,*,#8904,.T.);
#12206=ORIENTED_EDGE('',*,*,#8905,.T.);
#12207=ORIENTED_EDGE('',*,*,#8903,.F.);
#12208=ORIENTED_EDGE('',*,*,#8906,.T.);
#12209=ORIENTED_EDGE('',*,*,#8907,.T.);
#12210=ORIENTED_EDGE('',*,*,#8908,.T.);
#12211=ORIENTED_EDGE('',*,*,#8909,.T.);
#12212=ORIENTED_EDGE('',*,*,#8907,.F.);
#12213=ORIENTED_EDGE('',*,*,#8910,.T.);
#12214=ORIENTED_EDGE('',*,*,#8911,.T.);
#12215=ORIENTED_EDGE('',*,*,#8912,.T.);
#12216=ORIENTED_EDGE('',*,*,#8897,.F.);
#12217=ORIENTED_EDGE('',*,*,#8913,.F.);
#12218=ORIENTED_EDGE('',*,*,#8914,.F.);
#12219=ORIENTED_EDGE('',*,*,#8915,.T.);
#12220=ORIENTED_EDGE('',*,*,#8916,.T.);
#12221=ORIENTED_EDGE('',*,*,#8915,.F.);
#12222=ORIENTED_EDGE('',*,*,#8917,.F.);
#12223=ORIENTED_EDGE('',*,*,#8918,.F.);
#12224=ORIENTED_EDGE('',*,*,#8919,.T.);
#12225=ORIENTED_EDGE('',*,*,#8920,.T.);
#12226=ORIENTED_EDGE('',*,*,#8919,.F.);
#12227=ORIENTED_EDGE('',*,*,#8921,.T.);
#12228=ORIENTED_EDGE('',*,*,#8922,.T.);
#12229=ORIENTED_EDGE('',*,*,#8923,.T.);
#12230=ORIENTED_EDGE('',*,*,#8924,.T.);
#12231=ORIENTED_EDGE('',*,*,#8922,.F.);
#12232=ORIENTED_EDGE('',*,*,#8925,.T.);
#12233=ORIENTED_EDGE('',*,*,#8926,.T.);
#12234=ORIENTED_EDGE('',*,*,#8927,.T.);
#12235=ORIENTED_EDGE('',*,*,#8928,.T.);
#12236=ORIENTED_EDGE('',*,*,#8926,.F.);
#12237=ORIENTED_EDGE('',*,*,#8929,.F.);
#12238=ORIENTED_EDGE('',*,*,#8930,.F.);
#12239=ORIENTED_EDGE('',*,*,#8931,.T.);
#12240=ORIENTED_EDGE('',*,*,#8932,.T.);
#12241=ORIENTED_EDGE('',*,*,#8931,.F.);
#12242=ORIENTED_EDGE('',*,*,#8933,.F.);
#12243=ORIENTED_EDGE('',*,*,#8934,.F.);
#12244=ORIENTED_EDGE('',*,*,#8935,.T.);
#12245=ORIENTED_EDGE('',*,*,#8936,.T.);
#12246=ORIENTED_EDGE('',*,*,#8935,.F.);
#12247=ORIENTED_EDGE('',*,*,#8937,.T.);
#12248=ORIENTED_EDGE('',*,*,#8938,.T.);
#12249=ORIENTED_EDGE('',*,*,#8939,.T.);
#12250=ORIENTED_EDGE('',*,*,#8940,.T.);
#12251=ORIENTED_EDGE('',*,*,#8938,.F.);
#12252=ORIENTED_EDGE('',*,*,#8941,.F.);
#12253=ORIENTED_EDGE('',*,*,#8942,.F.);
#12254=ORIENTED_EDGE('',*,*,#8943,.T.);
#12255=ORIENTED_EDGE('',*,*,#8944,.T.);
#12256=ORIENTED_EDGE('',*,*,#8943,.F.);
#12257=ORIENTED_EDGE('',*,*,#8945,.T.);
#12258=ORIENTED_EDGE('',*,*,#8946,.T.);
#12259=ORIENTED_EDGE('',*,*,#8947,.T.);
#12260=ORIENTED_EDGE('',*,*,#8948,.T.);
#12261=ORIENTED_EDGE('',*,*,#8946,.F.);
#12262=ORIENTED_EDGE('',*,*,#8949,.F.);
#12263=ORIENTED_EDGE('',*,*,#8950,.F.);
#12264=ORIENTED_EDGE('',*,*,#8951,.T.);
#12265=ORIENTED_EDGE('',*,*,#8952,.T.);
#12266=ORIENTED_EDGE('',*,*,#8951,.F.);
#12267=ORIENTED_EDGE('',*,*,#8953,.T.);
#12268=ORIENTED_EDGE('',*,*,#8954,.T.);
#12269=ORIENTED_EDGE('',*,*,#8955,.T.);
#12270=ORIENTED_EDGE('',*,*,#8956,.T.);
#12271=ORIENTED_EDGE('',*,*,#8954,.F.);
#12272=ORIENTED_EDGE('',*,*,#8957,.F.);
#12273=ORIENTED_EDGE('',*,*,#8958,.F.);
#12274=ORIENTED_EDGE('',*,*,#8959,.T.);
#12275=ORIENTED_EDGE('',*,*,#8960,.T.);
#12276=ORIENTED_EDGE('',*,*,#8959,.F.);
#12277=ORIENTED_EDGE('',*,*,#8961,.T.);
#12278=ORIENTED_EDGE('',*,*,#8962,.T.);
#12279=ORIENTED_EDGE('',*,*,#8963,.T.);
#12280=ORIENTED_EDGE('',*,*,#8964,.T.);
#12281=ORIENTED_EDGE('',*,*,#8962,.F.);
#12282=ORIENTED_EDGE('',*,*,#8886,.T.);
#12283=ORIENTED_EDGE('',*,*,#8965,.T.);
#12284=ORIENTED_EDGE('',*,*,#8966,.T.);
#12285=ORIENTED_EDGE('',*,*,#8887,.F.);
#12286=ORIENTED_EDGE('',*,*,#8967,.T.);
#12287=ORIENTED_EDGE('',*,*,#8885,.T.);
#12288=ORIENTED_EDGE('',*,*,#8968,.T.);
#12289=ORIENTED_EDGE('',*,*,#8882,.T.);
#12290=ORIENTED_EDGE('',*,*,#8969,.T.);
#12291=ORIENTED_EDGE('',*,*,#8970,.T.);
#12292=ORIENTED_EDGE('',*,*,#8971,.T.);
#12293=ORIENTED_EDGE('',*,*,#8972,.T.);
#12294=ORIENTED_EDGE('',*,*,#8973,.T.);
#12295=ORIENTED_EDGE('',*,*,#8974,.T.);
#12296=ORIENTED_EDGE('',*,*,#8975,.T.);
#12297=ORIENTED_EDGE('',*,*,#8976,.F.);
#12298=ORIENTED_EDGE('',*,*,#8889,.F.);
#12299=ORIENTED_EDGE('',*,*,#8977,.F.);
#12300=ORIENTED_EDGE('',*,*,#8975,.F.);
#12301=ORIENTED_EDGE('',*,*,#8977,.T.);
#12302=ORIENTED_EDGE('',*,*,#8888,.F.);
#12303=ORIENTED_EDGE('',*,*,#8966,.F.);
#12304=ORIENTED_EDGE('',*,*,#8978,.F.);
#12305=ORIENTED_EDGE('',*,*,#8972,.F.);
#12306=ORIENTED_EDGE('',*,*,#8976,.T.);
#12307=ORIENTED_EDGE('',*,*,#8974,.F.);
#12308=ORIENTED_EDGE('',*,*,#8979,.F.);
#12309=ORIENTED_EDGE('',*,*,#8890,.F.);
#12310=ORIENTED_EDGE('',*,*,#8978,.T.);
#12311=ORIENTED_EDGE('',*,*,#8965,.F.);
#12312=ORIENTED_EDGE('',*,*,#8891,.F.);
#12313=ORIENTED_EDGE('',*,*,#8979,.T.);
#12314=ORIENTED_EDGE('',*,*,#8973,.F.);
#12315=ORIENTED_EDGE('',*,*,#8970,.F.);
#12316=ORIENTED_EDGE('',*,*,#8980,.T.);
#12317=ORIENTED_EDGE('',*,*,#8899,.F.);
#12318=ORIENTED_EDGE('',*,*,#8900,.F.);
#12319=ORIENTED_EDGE('',*,*,#8980,.F.);
#12320=ORIENTED_EDGE('',*,*,#8892,.F.);
#12321=ORIENTED_EDGE('',*,*,#8893,.F.);
#12322=ORIENTED_EDGE('',*,*,#8981,.T.);
#12323=ORIENTED_EDGE('',*,*,#8971,.F.);
#12324=ORIENTED_EDGE('',*,*,#8981,.F.);
#12325=ORIENTED_EDGE('',*,*,#8911,.F.);
#12326=ORIENTED_EDGE('',*,*,#8982,.T.);
#12327=ORIENTED_EDGE('',*,*,#8895,.F.);
#12328=ORIENTED_EDGE('',*,*,#8896,.F.);
#12329=ORIENTED_EDGE('',*,*,#8982,.F.);
#12330=ORIENTED_EDGE('',*,*,#8901,.F.);
#12331=ORIENTED_EDGE('',*,*,#8902,.F.);
#12332=ORIENTED_EDGE('',*,*,#8983,.T.);
#12333=ORIENTED_EDGE('',*,*,#8910,.F.);
#12334=ORIENTED_EDGE('',*,*,#8983,.F.);
#12335=ORIENTED_EDGE('',*,*,#8917,.T.);
#12336=ORIENTED_EDGE('',*,*,#8918,.T.);
#12337=ORIENTED_EDGE('',*,*,#8984,.T.);
#12338=ORIENTED_EDGE('',*,*,#8904,.F.);
#12339=ORIENTED_EDGE('',*,*,#8905,.F.);
#12340=ORIENTED_EDGE('',*,*,#8984,.F.);
#12341=ORIENTED_EDGE('',*,*,#8933,.T.);
#12342=ORIENTED_EDGE('',*,*,#8934,.T.);
#12343=ORIENTED_EDGE('',*,*,#8985,.T.);
#12344=ORIENTED_EDGE('',*,*,#8927,.F.);
#12345=ORIENTED_EDGE('',*,*,#8928,.F.);
#12346=ORIENTED_EDGE('',*,*,#8985,.F.);
#12347=ORIENTED_EDGE('',*,*,#8920,.F.);
#12348=ORIENTED_EDGE('',*,*,#8986,.T.);
#12349=ORIENTED_EDGE('',*,*,#8925,.F.);
#12350=ORIENTED_EDGE('',*,*,#8986,.F.);
#12351=ORIENTED_EDGE('',*,*,#8957,.T.);
#12352=ORIENTED_EDGE('',*,*,#8958,.T.);
#12353=ORIENTED_EDGE('',*,*,#8987,.T.);
#12354=ORIENTED_EDGE('',*,*,#8963,.F.);
#12355=ORIENTED_EDGE('',*,*,#8964,.F.);
#12356=ORIENTED_EDGE('',*,*,#8987,.F.);
#12357=ORIENTED_EDGE('',*,*,#8936,.F.);
#12358=ORIENTED_EDGE('',*,*,#8988,.T.);
#12359=ORIENTED_EDGE('',*,*,#8961,.F.);
#12360=ORIENTED_EDGE('',*,*,#8988,.F.);
#12361=ORIENTED_EDGE('',*,*,#8949,.T.);
#12362=ORIENTED_EDGE('',*,*,#8950,.T.);
#12363=ORIENTED_EDGE('',*,*,#8989,.T.);
#12364=ORIENTED_EDGE('',*,*,#8955,.F.);
#12365=ORIENTED_EDGE('',*,*,#8956,.F.);
#12366=ORIENTED_EDGE('',*,*,#8989,.F.);
#12367=ORIENTED_EDGE('',*,*,#8960,.F.);
#12368=ORIENTED_EDGE('',*,*,#8990,.T.);
#12369=ORIENTED_EDGE('',*,*,#8953,.F.);
#12370=ORIENTED_EDGE('',*,*,#8990,.F.);
#12371=ORIENTED_EDGE('',*,*,#8952,.F.);
#12372=ORIENTED_EDGE('',*,*,#8991,.T.);
#12373=ORIENTED_EDGE('',*,*,#8945,.F.);
#12374=ORIENTED_EDGE('',*,*,#8991,.F.);
#12375=ORIENTED_EDGE('',*,*,#8941,.T.);
#12376=ORIENTED_EDGE('',*,*,#8942,.T.);
#12377=ORIENTED_EDGE('',*,*,#8992,.T.);
#12378=ORIENTED_EDGE('',*,*,#8947,.F.);
#12379=ORIENTED_EDGE('',*,*,#8948,.F.);
#12380=ORIENTED_EDGE('',*,*,#8992,.F.);
#12381=ORIENTED_EDGE('',*,*,#8944,.F.);
#12382=ORIENTED_EDGE('',*,*,#8993,.T.);
#12383=ORIENTED_EDGE('',*,*,#8937,.F.);
#12384=ORIENTED_EDGE('',*,*,#8993,.F.);
#12385=ORIENTED_EDGE('',*,*,#8929,.T.);
#12386=ORIENTED_EDGE('',*,*,#8930,.T.);
#12387=ORIENTED_EDGE('',*,*,#8994,.T.);
#12388=ORIENTED_EDGE('',*,*,#8939,.F.);
#12389=ORIENTED_EDGE('',*,*,#8940,.F.);
#12390=ORIENTED_EDGE('',*,*,#8994,.F.);
#12391=ORIENTED_EDGE('',*,*,#8912,.F.);
#12392=ORIENTED_EDGE('',*,*,#8995,.T.);
#12393=ORIENTED_EDGE('',*,*,#8908,.F.);
#12394=ORIENTED_EDGE('',*,*,#8909,.F.);
#12395=ORIENTED_EDGE('',*,*,#8995,.F.);
#12396=ORIENTED_EDGE('',*,*,#8916,.F.);
#12397=ORIENTED_EDGE('',*,*,#8996,.T.);
#12398=ORIENTED_EDGE('',*,*,#8906,.F.);
#12399=ORIENTED_EDGE('',*,*,#8996,.F.);
#12400=ORIENTED_EDGE('',*,*,#8913,.T.);
#12401=ORIENTED_EDGE('',*,*,#8914,.T.);
#12402=ORIENTED_EDGE('',*,*,#8997,.T.);
#12403=ORIENTED_EDGE('',*,*,#8923,.F.);
#12404=ORIENTED_EDGE('',*,*,#8924,.F.);
#12405=ORIENTED_EDGE('',*,*,#8997,.F.);
#12406=ORIENTED_EDGE('',*,*,#8932,.F.);
#12407=ORIENTED_EDGE('',*,*,#8998,.T.);
#12408=ORIENTED_EDGE('',*,*,#8921,.F.);
#12409=ORIENTED_EDGE('',*,*,#8998,.F.);
#12410=ORIENTED_EDGE('',*,*,#8881,.T.);
#12411=ORIENTED_EDGE('',*,*,#8967,.F.);
#12412=ORIENTED_EDGE('',*,*,#8883,.F.);
#12413=ORIENTED_EDGE('',*,*,#8968,.F.);
#12414=ORIENTED_EDGE('',*,*,#8969,.F.);
#16557=PLANE('',#18413);
#16558=PLANE('',#18416);
#16559=PLANE('',#18470);
#16560=PLANE('',#18472);
#16561=PLANE('',#18474);
#16847=ADVANCED_FACE('',(#3731),#1530,.T.);
#16848=ADVANCED_FACE('',(#3732),#323,.T.);
#16849=ADVANCED_FACE('',(#3733),#3186,.F.);
#16850=ADVANCED_FACE('',(#3734),#3187,.T.);
#16851=ADVANCED_FACE('',(#3735),#3188,.T.);
#16852=ADVANCED_FACE('',(#3736),#3189,.T.);
#16853=ADVANCED_FACE('',(#3737,#3479),#16557,.F.);
#16854=ADVANCED_FACE('',(#3738,#3480),#16558,.T.);
#16855=ADVANCED_FACE('',(#3739),#3190,.T.);
#16856=ADVANCED_FACE('',(#3740),#3191,.T.);
#16857=ADVANCED_FACE('',(#3741),#3192,.T.);
#16858=ADVANCED_FACE('',(#3742),#3193,.T.);
#16859=ADVANCED_FACE('',(#3743),#3194,.T.);
#16860=ADVANCED_FACE('',(#3744),#3195,.T.);
#16861=ADVANCED_FACE('',(#3745),#3196,.T.);
#16862=ADVANCED_FACE('',(#3746),#3197,.T.);
#16863=ADVANCED_FACE('',(#3747),#3198,.T.);
#16864=ADVANCED_FACE('',(#3748),#3199,.T.);
#16865=ADVANCED_FACE('',(#3749),#3200,.T.);
#16866=ADVANCED_FACE('',(#3750),#3201,.T.);
#16867=ADVANCED_FACE('',(#3751),#3202,.T.);
#16868=ADVANCED_FACE('',(#3752),#324,.T.);
#16869=ADVANCED_FACE('',(#3753,#3481),#16559,.F.);
#16870=ADVANCED_FACE('',(#3754),#16560,.F.);
#16871=ADVANCED_FACE('',(#3755),#16561,.T.);
#16872=ADVANCED_FACE('',(#3756),#3203,.T.);
#16873=ADVANCED_FACE('',(#3757),#171,.T.);
#16874=ADVANCED_FACE('',(#3758),#172,.T.);
#16875=ADVANCED_FACE('',(#3759),#3204,.T.);
#16876=ADVANCED_FACE('',(#3760),#173,.F.);
#16877=ADVANCED_FACE('',(#3761),#174,.F.);
#16878=ADVANCED_FACE('',(#3762),#175,.T.);
#16879=ADVANCED_FACE('',(#3763),#176,.T.);
#16880=ADVANCED_FACE('',(#3764),#177,.T.);
#16881=ADVANCED_FACE('',(#3765),#178,.T.);
#16882=ADVANCED_FACE('',(#3766),#179,.T.);
#16883=ADVANCED_FACE('',(#3767),#180,.T.);
#16884=ADVANCED_FACE('',(#3768),#181,.T.);
#16885=ADVANCED_FACE('',(#3769),#182,.T.);
#16886=ADVANCED_FACE('',(#3770),#183,.T.);
#16887=ADVANCED_FACE('',(#3771),#184,.T.);
#16888=ADVANCED_FACE('',(#3772),#185,.T.);
#16889=ADVANCED_FACE('',(#3773),#186,.T.);
#16890=ADVANCED_FACE('',(#3774),#187,.T.);
#16891=ADVANCED_FACE('',(#3775),#188,.T.);
#16892=ADVANCED_FACE('',(#3776),#189,.T.);
#16893=ADVANCED_FACE('',(#3777),#190,.T.);
#16894=ADVANCED_FACE('',(#3778),#191,.T.);
#16895=ADVANCED_FACE('',(#3779),#1531,.T.);
#17667=CLOSED_SHELL('',(#16847,#16848,#16849,#16850,#16851,#16852,#16853,
#16854,#16855,#16856,#16857,#16858,#16859,#16860,#16861,#16862,#16863,#16864,
#16865,#16866,#16867,#16868,#16869,#16870,#16871,#16872,#16873,#16874,#16875,
#16876,#16877,#16878,#16879,#16880,#16881,#16882,#16883,#16884,#16885,#16886,
#16887,#16888,#16889,#16890,#16891,#16892,#16893,#16894,#16895));
#18394=AXIS2_PLACEMENT_3D('',#24840,#20904,#20905);
#18395=AXIS2_PLACEMENT_3D('',#25296,#20906,#20907);
#18396=AXIS2_PLACEMENT_3D('',#25299,#20908,#20909);
#18397=AXIS2_PLACEMENT_3D('',#25300,#20910,#20911);
#18398=AXIS2_PLACEMENT_3D('',#25304,#20913,#20914);
#18399=AXIS2_PLACEMENT_3D('',#25305,#20915,#20916);
#18400=AXIS2_PLACEMENT_3D('',#25306,#20917,#20918);
#18401=AXIS2_PLACEMENT_3D('',#25308,#20919,#20920);
#18402=AXIS2_PLACEMENT_3D('',#25312,#20922,#20923);
#18403=AXIS2_PLACEMENT_3D('',#25313,#20924,#20925);
#18404=AXIS2_PLACEMENT_3D('',#25314,#20926,#20927);
#18405=AXIS2_PLACEMENT_3D('',#25317,#20928,#20929);
#18406=AXIS2_PLACEMENT_3D('',#25318,#20930,#20931);
#18407=AXIS2_PLACEMENT_3D('',#25322,#20933,#20934);
#18408=AXIS2_PLACEMENT_3D('',#25323,#20935,#20936);
#18409=AXIS2_PLACEMENT_3D('',#25324,#20937,#20938);
#18410=AXIS2_PLACEMENT_3D('',#25326,#20939,#20940);
#18411=AXIS2_PLACEMENT_3D('',#25330,#20942,#20943);
#18412=AXIS2_PLACEMENT_3D('',#25331,#20944,#20945);
#18413=AXIS2_PLACEMENT_3D('',#25332,#20946,#20947);
#18414=AXIS2_PLACEMENT_3D('',#25334,#20948,#20949);
#18415=AXIS2_PLACEMENT_3D('',#25336,#20950,#20951);
#18416=AXIS2_PLACEMENT_3D('',#25337,#20952,#20953);
#18417=AXIS2_PLACEMENT_3D('',#25339,#20954,#20955);
#18418=AXIS2_PLACEMENT_3D('',#25340,#20956,#20957);
#18419=AXIS2_PLACEMENT_3D('',#25343,#20958,#20959);
#18420=AXIS2_PLACEMENT_3D('',#25344,#20960,#20961);
#18421=AXIS2_PLACEMENT_3D('',#25347,#20963,#20964);
#18422=AXIS2_PLACEMENT_3D('',#25348,#20965,#20966);
#18423=AXIS2_PLACEMENT_3D('',#25351,#20967,#20968);
#18424=AXIS2_PLACEMENT_3D('',#25352,#20969,#20970);
#18425=AXIS2_PLACEMENT_3D('',#25355,#20972,#20973);
#18426=AXIS2_PLACEMENT_3D('',#25356,#20974,#20975);
#18427=AXIS2_PLACEMENT_3D('',#25358,#20976,#20977);
#18428=AXIS2_PLACEMENT_3D('',#25362,#20979,#20980);
#18429=AXIS2_PLACEMENT_3D('',#25363,#20981,#20982);
#18430=AXIS2_PLACEMENT_3D('',#25364,#20983,#20984);
#18431=AXIS2_PLACEMENT_3D('',#25366,#20985,#20986);
#18432=AXIS2_PLACEMENT_3D('',#25370,#20988,#20989);
#18433=AXIS2_PLACEMENT_3D('',#25371,#20990,#20991);
#18434=AXIS2_PLACEMENT_3D('',#25372,#20992,#20993);
#18435=AXIS2_PLACEMENT_3D('',#25375,#20994,#20995);
#18436=AXIS2_PLACEMENT_3D('',#25376,#20996,#20997);
#18437=AXIS2_PLACEMENT_3D('',#25379,#20999,#21000);
#18438=AXIS2_PLACEMENT_3D('',#25380,#21001,#21002);
#18439=AXIS2_PLACEMENT_3D('',#25383,#21003,#21004);
#18440=AXIS2_PLACEMENT_3D('',#25384,#21005,#21006);
#18441=AXIS2_PLACEMENT_3D('',#25387,#21008,#21009);
#18442=AXIS2_PLACEMENT_3D('',#25388,#21010,#21011);
#18443=AXIS2_PLACEMENT_3D('',#25390,#21012,#21013);
#18444=AXIS2_PLACEMENT_3D('',#25394,#21015,#21016);
#18445=AXIS2_PLACEMENT_3D('',#25395,#21017,#21018);
#18446=AXIS2_PLACEMENT_3D('',#25396,#21019,#21020);
#18447=AXIS2_PLACEMENT_3D('',#25399,#21021,#21022);
#18448=AXIS2_PLACEMENT_3D('',#25400,#21023,#21024);
#18449=AXIS2_PLACEMENT_3D('',#25403,#21026,#21027);
#18450=AXIS2_PLACEMENT_3D('',#25404,#21028,#21029);
#18451=AXIS2_PLACEMENT_3D('',#25406,#21030,#21031);
#18452=AXIS2_PLACEMENT_3D('',#25410,#21033,#21034);
#18453=AXIS2_PLACEMENT_3D('',#25411,#21035,#21036);
#18454=AXIS2_PLACEMENT_3D('',#25412,#21037,#21038);
#18455=AXIS2_PLACEMENT_3D('',#25415,#21039,#21040);
#18456=AXIS2_PLACEMENT_3D('',#25416,#21041,#21042);
#18457=AXIS2_PLACEMENT_3D('',#25419,#21044,#21045);
#18458=AXIS2_PLACEMENT_3D('',#25420,#21046,#21047);
#18459=AXIS2_PLACEMENT_3D('',#25422,#21048,#21049);
#18460=AXIS2_PLACEMENT_3D('',#25426,#21051,#21052);
#18461=AXIS2_PLACEMENT_3D('',#25427,#21053,#21054);
#18462=AXIS2_PLACEMENT_3D('',#25428,#21055,#21056);
#18463=AXIS2_PLACEMENT_3D('',#25431,#21057,#21058);
#18464=AXIS2_PLACEMENT_3D('',#25432,#21059,#21060);
#18465=AXIS2_PLACEMENT_3D('',#25435,#21062,#21063);
#18466=AXIS2_PLACEMENT_3D('',#25436,#21064,#21065);
#18467=AXIS2_PLACEMENT_3D('',#25438,#21066,#21067);
#18468=AXIS2_PLACEMENT_3D('',#25442,#21069,#21070);
#18469=AXIS2_PLACEMENT_3D('',#25443,#21071,#21072);
#18470=AXIS2_PLACEMENT_3D('',#25544,#21073,#21074);
#18471=AXIS2_PLACEMENT_3D('',#25555,#21075,#21076);
#18472=AXIS2_PLACEMENT_3D('',#25556,#21077,#21078);
#18473=AXIS2_PLACEMENT_3D('',#25558,#21079,#21080);
#18474=AXIS2_PLACEMENT_3D('',#25559,#21081,#21082);
#18475=AXIS2_PLACEMENT_3D('',#25688,#21083,#21084);
#18476=AXIS2_PLACEMENT_3D('',#25715,#21085,#21086);
#18477=AXIS2_PLACEMENT_3D('',#25729,#21087,#21088);
#18478=AXIS2_PLACEMENT_3D('',#25743,#21089,#21090);
#18479=AXIS2_PLACEMENT_3D('',#25744,#21091,#21092);
#18480=AXIS2_PLACEMENT_3D('',#25745,#21093,#21094);
#18481=AXIS2_PLACEMENT_3D('',#25746,#21095,#21096);
#18482=AXIS2_PLACEMENT_3D('',#25747,#21097,#21098);
#18483=AXIS2_PLACEMENT_3D('',#25748,#21099,#21100);
#18484=AXIS2_PLACEMENT_3D('',#25749,#21101,#21102);
#18485=AXIS2_PLACEMENT_3D('',#25750,#21103,#21104);
#18486=AXIS2_PLACEMENT_3D('',#25751,#21105,#21106);
#18487=AXIS2_PLACEMENT_3D('',#25752,#21107,#21108);
#18488=AXIS2_PLACEMENT_3D('',#25753,#21109,#21110);
#18489=AXIS2_PLACEMENT_3D('',#25754,#21111,#21112);
#18490=AXIS2_PLACEMENT_3D('',#25755,#21113,#21114);
#18491=AXIS2_PLACEMENT_3D('',#25756,#21115,#21116);
#18492=AXIS2_PLACEMENT_3D('',#25757,#21117,#21118);
#18493=AXIS2_PLACEMENT_3D('',#25758,#21119,#21120);
#18494=AXIS2_PLACEMENT_3D('',#25759,#21121,#21122);
#18495=AXIS2_PLACEMENT_3D('',#25760,#21123,#21124);
#18496=AXIS2_PLACEMENT_3D('',#25761,#21125,#21126);
#18497=AXIS2_PLACEMENT_3D('',#25762,#21127,#21128);
#18498=AXIS2_PLACEMENT_3D('',#25763,#21129,#21130);
#18499=AXIS2_PLACEMENT_3D('',#25764,#21131,#21132);
#18500=AXIS2_PLACEMENT_3D('',#25765,#21133,#21134);
#18501=AXIS2_PLACEMENT_3D('',#25766,#21135,#21136);
#18502=AXIS2_PLACEMENT_3D('',#25767,#21137,#21138);
#18503=AXIS2_PLACEMENT_3D('',#25768,#21139,#21140);
#18504=AXIS2_PLACEMENT_3D('',#25769,#21141,#21142);
#18505=AXIS2_PLACEMENT_3D('',#25770,#21143,#21144);
#18506=AXIS2_PLACEMENT_3D('',#25771,#21145,#21146);
#18507=AXIS2_PLACEMENT_3D('',#25772,#21147,#21148);
#18508=AXIS2_PLACEMENT_3D('',#25773,#21149,#21150);
#18509=AXIS2_PLACEMENT_3D('',#25774,#21151,#21152);
#18510=AXIS2_PLACEMENT_3D('',#25775,#21153,#21154);
#18511=AXIS2_PLACEMENT_3D('',#25776,#21155,#21156);
#18512=AXIS2_PLACEMENT_3D('',#25777,#21157,#21158);
#18513=AXIS2_PLACEMENT_3D('',#25778,#21159,#21160);
#18514=AXIS2_PLACEMENT_3D('',#25779,#21161,#21162);
#18515=AXIS2_PLACEMENT_3D('',#25780,#21163,#21164);
#18516=AXIS2_PLACEMENT_3D('',#25781,#21165,#21166);
#20904=DIRECTION('axis',(0.,0.,1.));
#20905=DIRECTION('refdir',(1.,0.,0.));
#20906=DIRECTION('center_axis',(1.,0.,0.));
#20907=DIRECTION('ref_axis',(0.,0.,-1.));
#20908=DIRECTION('center_axis',(-1.,0.,0.));
#20909=DIRECTION('ref_axis',(0.,0.,1.));
#20910=DIRECTION('center_axis',(-1.,0.,0.));
#20911=DIRECTION('ref_axis',(0.,0.,1.));
#20912=DIRECTION('',(1.,0.,0.));
#20913=DIRECTION('center_axis',(-1.,0.,0.));
#20914=DIRECTION('ref_axis',(0.,0.,1.));
#20915=DIRECTION('center_axis',(-1.,0.,0.));
#20916=DIRECTION('ref_axis',(0.,0.,1.));
#20917=DIRECTION('center_axis',(1.,0.,0.));
#20918=DIRECTION('ref_axis',(0.,0.,-1.));
#20919=DIRECTION('center_axis',(-1.,0.,0.));
#20920=DIRECTION('ref_axis',(0.,0.,1.));
#20921=DIRECTION('',(-1.,0.,0.));
#20922=DIRECTION('center_axis',(-1.,0.,0.));
#20923=DIRECTION('ref_axis',(0.,0.,1.));
#20924=DIRECTION('center_axis',(-1.,0.,0.));
#20925=DIRECTION('ref_axis',(0.,0.,1.));
#20926=DIRECTION('center_axis',(1.,0.,0.));
#20927=DIRECTION('ref_axis',(0.,0.,-1.));
#20928=DIRECTION('center_axis',(-1.,0.,0.));
#20929=DIRECTION('ref_axis',(0.,0.,1.));
#20930=DIRECTION('center_axis',(-1.,0.,0.));
#20931=DIRECTION('ref_axis',(0.,0.,1.));
#20932=DIRECTION('',(-1.,0.,0.));
#20933=DIRECTION('center_axis',(-1.,0.,0.));
#20934=DIRECTION('ref_axis',(0.,0.,1.));
#20935=DIRECTION('center_axis',(-1.,0.,0.));
#20936=DIRECTION('ref_axis',(0.,0.,1.));
#20937=DIRECTION('center_axis',(1.,0.,0.));
#20938=DIRECTION('ref_axis',(0.,0.,-1.));
#20939=DIRECTION('center_axis',(1.,0.,0.));
#20940=DIRECTION('ref_axis',(0.,0.,-1.));
#20941=DIRECTION('',(-1.,0.,0.));
#20942=DIRECTION('center_axis',(-1.,0.,0.));
#20943=DIRECTION('ref_axis',(0.,0.,1.));
#20944=DIRECTION('center_axis',(-1.,0.,0.));
#20945=DIRECTION('ref_axis',(0.,0.,1.));
#20946=DIRECTION('center_axis',(-1.,0.,0.));
#20947=DIRECTION('ref_axis',(0.,0.,1.));
#20948=DIRECTION('center_axis',(-1.,0.,0.));
#20949=DIRECTION('ref_axis',(0.,0.,1.));
#20950=DIRECTION('center_axis',(-1.,0.,0.));
#20951=DIRECTION('ref_axis',(0.,0.,1.));
#20952=DIRECTION('center_axis',(-1.,0.,0.));
#20953=DIRECTION('ref_axis',(0.,0.,1.));
#20954=DIRECTION('center_axis',(-1.,0.,0.));
#20955=DIRECTION('ref_axis',(0.,0.,1.));
#20956=DIRECTION('center_axis',(1.,0.,0.));
#20957=DIRECTION('ref_axis',(0.,0.,-1.));
#20958=DIRECTION('center_axis',(1.,0.,0.));
#20959=DIRECTION('ref_axis',(0.,0.,-1.));
#20960=DIRECTION('center_axis',(1.,0.,0.));
#20961=DIRECTION('ref_axis',(0.,0.,-1.));
#20962=DIRECTION('',(-1.,0.,0.));
#20963=DIRECTION('center_axis',(1.,0.,0.));
#20964=DIRECTION('ref_axis',(0.,0.,-1.));
#20965=DIRECTION('center_axis',(1.,0.,0.));
#20966=DIRECTION('ref_axis',(0.,0.,-1.));
#20967=DIRECTION('center_axis',(1.,0.,0.));
#20968=DIRECTION('ref_axis',(0.,0.,-1.));
#20969=DIRECTION('center_axis',(1.,0.,0.));
#20970=DIRECTION('ref_axis',(0.,0.,-1.));
#20971=DIRECTION('',(-1.,0.,0.));
#20972=DIRECTION('center_axis',(1.,0.,0.));
#20973=DIRECTION('ref_axis',(0.,0.,-1.));
#20974=DIRECTION('center_axis',(1.,0.,0.));
#20975=DIRECTION('ref_axis',(0.,0.,-1.));
#20976=DIRECTION('center_axis',(1.,0.,0.));
#20977=DIRECTION('ref_axis',(0.,0.,-1.));
#20978=DIRECTION('',(-1.,0.,0.));
#20979=DIRECTION('center_axis',(-1.,0.,0.));
#20980=DIRECTION('ref_axis',(0.,0.,1.));
#20981=DIRECTION('center_axis',(-1.,0.,0.));
#20982=DIRECTION('ref_axis',(0.,0.,1.));
#20983=DIRECTION('center_axis',(1.,0.,0.));
#20984=DIRECTION('ref_axis',(0.,0.,-1.));
#20985=DIRECTION('center_axis',(1.,0.,0.));
#20986=DIRECTION('ref_axis',(0.,0.,-1.));
#20987=DIRECTION('',(-1.,0.,0.));
#20988=DIRECTION('center_axis',(-1.,0.,0.));
#20989=DIRECTION('ref_axis',(0.,0.,1.));
#20990=DIRECTION('center_axis',(-1.,0.,0.));
#20991=DIRECTION('ref_axis',(0.,0.,1.));
#20992=DIRECTION('center_axis',(1.,0.,0.));
#20993=DIRECTION('ref_axis',(0.,0.,-1.));
#20994=DIRECTION('center_axis',(1.,0.,0.));
#20995=DIRECTION('ref_axis',(0.,0.,-1.));
#20996=DIRECTION('center_axis',(1.,0.,0.));
#20997=DIRECTION('ref_axis',(0.,0.,-1.));
#20998=DIRECTION('',(-1.,0.,0.));
#20999=DIRECTION('center_axis',(1.,0.,0.));
#21000=DIRECTION('ref_axis',(0.,0.,-1.));
#21001=DIRECTION('center_axis',(1.,0.,0.));
#21002=DIRECTION('ref_axis',(0.,0.,-1.));
#21003=DIRECTION('center_axis',(1.,0.,0.));
#21004=DIRECTION('ref_axis',(0.,0.,-1.));
#21005=DIRECTION('center_axis',(1.,0.,0.));
#21006=DIRECTION('ref_axis',(0.,0.,-1.));
#21007=DIRECTION('',(-1.,0.,0.));
#21008=DIRECTION('center_axis',(1.,0.,0.));
#21009=DIRECTION('ref_axis',(0.,0.,-1.));
#21010=DIRECTION('center_axis',(1.,0.,0.));
#21011=DIRECTION('ref_axis',(0.,0.,-1.));
#21012=DIRECTION('center_axis',(1.,0.,0.));
#21013=DIRECTION('ref_axis',(0.,0.,-1.));
#21014=DIRECTION('',(-1.,0.,0.));
#21015=DIRECTION('center_axis',(-1.,0.,0.));
#21016=DIRECTION('ref_axis',(0.,0.,1.));
#21017=DIRECTION('center_axis',(-1.,0.,0.));
#21018=DIRECTION('ref_axis',(0.,0.,1.));
#21019=DIRECTION('center_axis',(1.,0.,0.));
#21020=DIRECTION('ref_axis',(0.,0.,-1.));
#21021=DIRECTION('center_axis',(1.,0.,0.));
#21022=DIRECTION('ref_axis',(0.,0.,-1.));
#21023=DIRECTION('center_axis',(1.,0.,0.));
#21024=DIRECTION('ref_axis',(0.,0.,-1.));
#21025=DIRECTION('',(-1.,0.,0.));
#21026=DIRECTION('center_axis',(1.,0.,0.));
#21027=DIRECTION('ref_axis',(0.,0.,-1.));
#21028=DIRECTION('center_axis',(1.,0.,0.));
#21029=DIRECTION('ref_axis',(0.,0.,-1.));
#21030=DIRECTION('center_axis',(1.,0.,0.));
#21031=DIRECTION('ref_axis',(0.,0.,-1.));
#21032=DIRECTION('',(-1.,0.,0.));
#21033=DIRECTION('center_axis',(-1.,0.,0.));
#21034=DIRECTION('ref_axis',(0.,0.,1.));
#21035=DIRECTION('center_axis',(-1.,0.,0.));
#21036=DIRECTION('ref_axis',(0.,0.,1.));
#21037=DIRECTION('center_axis',(1.,0.,0.));
#21038=DIRECTION('ref_axis',(0.,0.,-1.));
#21039=DIRECTION('center_axis',(1.,0.,0.));
#21040=DIRECTION('ref_axis',(0.,0.,-1.));
#21041=DIRECTION('center_axis',(1.,0.,0.));
#21042=DIRECTION('ref_axis',(0.,0.,-1.));
#21043=DIRECTION('',(-1.,0.,0.));
#21044=DIRECTION('center_axis',(1.,0.,0.));
#21045=DIRECTION('ref_axis',(0.,0.,-1.));
#21046=DIRECTION('center_axis',(1.,0.,0.));
#21047=DIRECTION('ref_axis',(0.,0.,-1.));
#21048=DIRECTION('center_axis',(1.,0.,0.));
#21049=DIRECTION('ref_axis',(0.,0.,-1.));
#21050=DIRECTION('',(-1.,0.,0.));
#21051=DIRECTION('center_axis',(-1.,0.,0.));
#21052=DIRECTION('ref_axis',(0.,0.,1.));
#21053=DIRECTION('center_axis',(-1.,0.,0.));
#21054=DIRECTION('ref_axis',(0.,0.,1.));
#21055=DIRECTION('center_axis',(1.,0.,0.));
#21056=DIRECTION('ref_axis',(0.,0.,-1.));
#21057=DIRECTION('center_axis',(1.,0.,0.));
#21058=DIRECTION('ref_axis',(0.,0.,-1.));
#21059=DIRECTION('center_axis',(1.,0.,0.));
#21060=DIRECTION('ref_axis',(0.,0.,-1.));
#21061=DIRECTION('',(-1.,0.,0.));
#21062=DIRECTION('center_axis',(1.,0.,0.));
#21063=DIRECTION('ref_axis',(0.,0.,-1.));
#21064=DIRECTION('center_axis',(1.,0.,0.));
#21065=DIRECTION('ref_axis',(0.,0.,-1.));
#21066=DIRECTION('center_axis',(1.,0.,0.));
#21067=DIRECTION('ref_axis',(0.,0.,-1.));
#21068=DIRECTION('',(-1.,0.,0.));
#21069=DIRECTION('center_axis',(-1.,0.,0.));
#21070=DIRECTION('ref_axis',(0.,0.,1.));
#21071=DIRECTION('center_axis',(-1.,0.,0.));
#21072=DIRECTION('ref_axis',(0.,0.,1.));
#21073=DIRECTION('center_axis',(-1.,0.,0.));
#21074=DIRECTION('ref_axis',(0.,0.,1.));
#21075=DIRECTION('center_axis',(-1.,0.,0.));
#21076=DIRECTION('ref_axis',(0.,0.,1.));
#21077=DIRECTION('center_axis',(-1.,0.,0.));
#21078=DIRECTION('ref_axis',(0.,0.,1.));
#21079=DIRECTION('center_axis',(-1.,0.,0.));
#21080=DIRECTION('ref_axis',(0.,0.,1.));
#21081=DIRECTION('center_axis',(-1.,0.,0.));
#21082=DIRECTION('ref_axis',(0.,0.,1.));
#21083=DIRECTION('center_axis',(-5.01652904731627E-15,2.04600742668907E-13,
1.));
#21084=DIRECTION('ref_axis',(0.,-1.,2.04600742668907E-13));
#21085=DIRECTION('center_axis',(0.999999999999512,3.64455443991191E-10,
9.88227092522604E-7));
#21086=DIRECTION('ref_axis',(-9.88227091978951E-7,2.02026683180761E-10,
0.999999999999512));
#21087=DIRECTION('center_axis',(0.999999999999512,-3.64455669902473E-10,
-9.88227186270797E-7));
#21088=DIRECTION('ref_axis',(-9.88227185993996E-7,0.,-0.999999999999512));
#21089=DIRECTION('center_axis',(3.96697174057741E-14,2.06573350065547E-12,
1.));
#21090=DIRECTION('ref_axis',(0.,-1.,2.06573350065547E-12));
#21091=DIRECTION('center_axis',(-1.,0.,0.));
#21092=DIRECTION('ref_axis',(0.,0.,1.));
#21093=DIRECTION('center_axis',(0.,1.,-1.30989755110808E-16));
#21094=DIRECTION('ref_axis',(0.,-1.30989755110808E-16,-1.));
#21095=DIRECTION('center_axis',(-1.,0.,0.));
#21096=DIRECTION('ref_axis',(0.,0.,1.));
#21097=DIRECTION('center_axis',(0.,1.,-2.22044604925031E-16));
#21098=DIRECTION('ref_axis',(0.,-2.22044604925031E-16,-1.));
#21099=DIRECTION('center_axis',(-1.,0.,0.));
#21100=DIRECTION('ref_axis',(0.,0.,1.));
#21101=DIRECTION('center_axis',(0.,-1.,1.85037170770859E-16));
#21102=DIRECTION('ref_axis',(0.,-1.85037170770859E-16,-1.));
#21103=DIRECTION('center_axis',(-1.,0.,0.));
#21104=DIRECTION('ref_axis',(0.,0.,1.));
#21105=DIRECTION('center_axis',(0.,-1.,1.19009136371855E-16));
#21106=DIRECTION('ref_axis',(0.,-1.19009136371855E-16,-1.));
#21107=DIRECTION('center_axis',(-1.,0.,0.));
#21108=DIRECTION('ref_axis',(0.,0.,1.));
#21109=DIRECTION('center_axis',(0.,-1.,1.19009136371855E-16));
#21110=DIRECTION('ref_axis',(0.,-1.19009136371855E-16,-1.));
#21111=DIRECTION('center_axis',(-1.,0.,0.));
#21112=DIRECTION('ref_axis',(0.,0.,1.));
#21113=DIRECTION('center_axis',(0.,-1.,1.19009136371855E-16));
#21114=DIRECTION('ref_axis',(0.,-1.19009136371855E-16,-1.));
#21115=DIRECTION('center_axis',(1.,0.,0.));
#21116=DIRECTION('ref_axis',(0.,0.,-1.));
#21117=DIRECTION('center_axis',(0.,-1.,-1.19009136371855E-16));
#21118=DIRECTION('ref_axis',(0.,-1.19009136371855E-16,1.));
#21119=DIRECTION('center_axis',(-1.,0.,0.));
#21120=DIRECTION('ref_axis',(0.,0.,1.));
#21121=DIRECTION('center_axis',(0.,-1.,1.19009136371855E-16));
#21122=DIRECTION('ref_axis',(0.,-1.19009136371855E-16,-1.));
#21123=DIRECTION('center_axis',(1.,0.,0.));
#21124=DIRECTION('ref_axis',(0.,0.,-1.));
#21125=DIRECTION('center_axis',(0.,-1.,-1.19009136371855E-16));
#21126=DIRECTION('ref_axis',(0.,-1.19009136371855E-16,1.));
#21127=DIRECTION('center_axis',(-1.,0.,0.));
#21128=DIRECTION('ref_axis',(0.,0.,1.));
#21129=DIRECTION('center_axis',(0.,-1.,1.19009136371855E-16));
#21130=DIRECTION('ref_axis',(0.,-1.19009136371855E-16,-1.));
#21131=DIRECTION('center_axis',(1.,0.,0.));
#21132=DIRECTION('ref_axis',(0.,0.,-1.));
#21133=DIRECTION('center_axis',(0.,-1.,-1.19009136371855E-16));
#21134=DIRECTION('ref_axis',(0.,-1.19009136371855E-16,1.));
#21135=DIRECTION('center_axis',(1.,0.,0.));
#21136=DIRECTION('ref_axis',(0.,0.,-1.));
#21137=DIRECTION('center_axis',(0.,-1.,-1.19009136371855E-16));
#21138=DIRECTION('ref_axis',(0.,-1.19009136371855E-16,1.));
#21139=DIRECTION('center_axis',(-1.,0.,0.));
#21140=DIRECTION('ref_axis',(0.,0.,1.));
#21141=DIRECTION('center_axis',(0.,-1.,1.19009136371855E-16));
#21142=DIRECTION('ref_axis',(0.,-1.19009136371855E-16,-1.));
#21143=DIRECTION('center_axis',(1.,0.,0.));
#21144=DIRECTION('ref_axis',(0.,0.,-1.));
#21145=DIRECTION('center_axis',(0.,-1.,-1.19009136371855E-16));
#21146=DIRECTION('ref_axis',(0.,-1.19009136371855E-16,1.));
#21147=DIRECTION('center_axis',(-1.,0.,0.));
#21148=DIRECTION('ref_axis',(0.,0.,1.));
#21149=DIRECTION('center_axis',(0.,-1.,1.19009136371855E-16));
#21150=DIRECTION('ref_axis',(0.,-1.19009136371855E-16,-1.));
#21151=DIRECTION('center_axis',(-1.,0.,0.));
#21152=DIRECTION('ref_axis',(0.,0.,1.));
#21153=DIRECTION('center_axis',(0.,-1.,1.19009136371855E-16));
#21154=DIRECTION('ref_axis',(0.,-1.19009136371855E-16,-1.));
#21155=DIRECTION('center_axis',(1.,0.,0.));
#21156=DIRECTION('ref_axis',(0.,0.,-1.));
#21157=DIRECTION('center_axis',(0.,-1.,-1.19009136371855E-16));
#21158=DIRECTION('ref_axis',(0.,-1.19009136371855E-16,1.));
#21159=DIRECTION('center_axis',(-1.,0.,0.));
#21160=DIRECTION('ref_axis',(0.,0.,1.));
#21161=DIRECTION('center_axis',(0.,-1.,1.19009136371855E-16));
#21162=DIRECTION('ref_axis',(0.,-1.19009136371855E-16,-1.));
#21163=DIRECTION('center_axis',(1.,0.,0.));
#21164=DIRECTION('ref_axis',(0.,0.,-1.));
#21165=DIRECTION('center_axis',(0.,-1.,-1.19009136371855E-16));
#21166=DIRECTION('ref_axis',(0.,-1.19009136371855E-16,1.));
#24840=CARTESIAN_POINT('',(0.,0.,0.));
#24841=CARTESIAN_POINT('Ctrl Pts',(-0.180492715511507,0.00208357847138839,
0.00778381458262853));
#24842=CARTESIAN_POINT('Ctrl Pts',(-0.18,0.00208768551873161,0.00777792629190908));
#24843=CARTESIAN_POINT('Ctrl Pts',(-0.18,0.00236958913814357,0.00737375990977421));
#24844=CARTESIAN_POINT('Ctrl Pts',(-0.180494324020048,0.00106537901854582,
0.00707337168038232));
#24845=CARTESIAN_POINT('Ctrl Pts',(-0.18,0.00106751218715109,0.00706776299687777));
#24846=CARTESIAN_POINT('Ctrl Pts',(-0.18,0.0014052360688775,0.00670086601600097));
#24847=CARTESIAN_POINT('Ctrl Pts',(-0.180498282439035,-0.000688149212900568,
0.00524596704164286));
#24848=CARTESIAN_POINT('Ctrl Pts',(-0.18,-0.000692161918799494,0.00523579826232968));
#24849=CARTESIAN_POINT('Ctrl Pts',(-0.18,-0.000255396373108266,0.00497022946835977));
#24850=CARTESIAN_POINT('Ctrl Pts',(-0.180508571884256,-0.00206121245391611,
0.00171196042612565));
#24851=CARTESIAN_POINT('Ctrl Pts',(-0.18,-0.00207089065980965,0.0017061119940659));
#24852=CARTESIAN_POINT('Ctrl Pts',(-0.18,-0.00155636923028695,0.001622484125152));
#24853=CARTESIAN_POINT('Ctrl Pts',(-0.180507701632299,-0.00198984920249958,
-0.00207534072170255));
#24854=CARTESIAN_POINT('Ctrl Pts',(-0.18,-0.00199898872775875,-0.00206848014615668));
#24855=CARTESIAN_POINT('Ctrl Pts',(-0.18,-0.0014886043286521,-0.00196703616742313));
#24856=CARTESIAN_POINT('Ctrl Pts',(-0.180497559880866,-0.000482912630366871,
-0.00555392798696781));
#24857=CARTESIAN_POINT('Ctrl Pts',(-0.18,-0.000486526972169703,-0.00554405840433583));
#24858=CARTESIAN_POINT('Ctrl Pts',(-0.18,-6.11665353613021E-5,-0.00526163542994926));
#24859=CARTESIAN_POINT('Ctrl Pts',(-0.180491867056987,0.00224576313070539,
-0.0081898374281038));
#24860=CARTESIAN_POINT('Ctrl Pts',(-0.18,0.00224601031558402,-0.00818083867958575));
#24861=CARTESIAN_POINT('Ctrl Pts',(-0.18,0.00252313449484398,-0.00775830380791825));
#24862=CARTESIAN_POINT('Ctrl Pts',(-0.180488462887617,0.00577942932125372,
-0.00958054386633694));
#24863=CARTESIAN_POINT('Ctrl Pts',(-0.18,0.00577937831377157,-0.00956893262499887));
#24864=CARTESIAN_POINT('Ctrl Pts',(-0.18,0.00587025317906997,-0.00907572435223234));
#24865=CARTESIAN_POINT('Ctrl Pts',(-0.180488629342552,0.00957710911122243,
-0.00950944489475148));
#24866=CARTESIAN_POINT('Ctrl Pts',(-0.18,0.00957712259305036,-0.00949788380666547));
#24867=CARTESIAN_POINT('Ctrl Pts',(-0.18,0.0094675316846421,-0.00900837007444288));
#24868=CARTESIAN_POINT('Ctrl Pts',(-0.180492343722264,0.0130567083237039,
-0.00798771374964044));
#24869=CARTESIAN_POINT('Ctrl Pts',(-0.18,0.0130566470856787,-0.00797903414015096));
#24870=CARTESIAN_POINT('Ctrl Pts',(-0.18,0.0127633603172519,-0.00756679005675688));
#24871=CARTESIAN_POINT('Ctrl Pts',(-0.180498277776074,0.0156878479525759,
-0.00524728696109442));
#24872=CARTESIAN_POINT('Ctrl Pts',(-0.18,0.0156918696359066,-0.00523708434816095));
#24873=CARTESIAN_POINT('Ctrl Pts',(-0.18,0.0152551103542225,-0.00497147978047479));
#24874=CARTESIAN_POINT('Ctrl Pts',(-0.180508590057067,0.0170631420237172,
-0.00170670572622402));
#24875=CARTESIAN_POINT('Ctrl Pts',(-0.18,0.0170728417288127,-0.00170085628138549));
#24876=CARTESIAN_POINT('Ctrl Pts',(-0.18,0.0165581992152197,-0.00161750652259339));
#24877=CARTESIAN_POINT('Ctrl Pts',(-0.180507676294974,0.0169879516360366,
0.00208672420876621));
#24878=CARTESIAN_POINT('Ctrl Pts',(-0.18,0.0169970776392087,0.00207981994539201));
#24879=CARTESIAN_POINT('Ctrl Pts',(-0.18,0.0164868018720009,0.00197783354485042));
#24880=CARTESIAN_POINT('Ctrl Pts',(-0.180497532146321,0.0154750030588555,
0.00556552633006958));
#24881=CARTESIAN_POINT('Ctrl Pts',(-0.18,0.0154786081176936,0.00555565825322737));
#24882=CARTESIAN_POINT('Ctrl Pts',(-0.18,0.0150536805229185,0.00527261080601529));
#24883=CARTESIAN_POINT('Ctrl Pts',(-0.180491851706073,0.0127430969971975,
0.00819641820051746));
#24884=CARTESIAN_POINT('Ctrl Pts',(-0.18,0.0127428333825127,0.00818741797918455));
#24885=CARTESIAN_POINT('Ctrl Pts',(-0.18,0.01246631245657,0.00776454042759482));
#24886=CARTESIAN_POINT('Ctrl Pts',(-0.180488461754297,0.00921325615876769,
0.00958099954636007));
#24887=CARTESIAN_POINT('Ctrl Pts',(-0.18,0.00921330243936221,0.00956938959009847));
#24888=CARTESIAN_POINT('Ctrl Pts',(-0.18,0.00912281682762101,0.00907615564159787));
#24889=CARTESIAN_POINT('Ctrl Pts',(-0.18048863138779,0.00542104750415485,
0.00950862445512012));
#24890=CARTESIAN_POINT('Ctrl Pts',(-0.18,0.00542103959480098,0.00949706815102514));
#24891=CARTESIAN_POINT('Ctrl Pts',(-0.18,0.00553072204248816,0.00900759283099922));
#24892=CARTESIAN_POINT('Ctrl Pts',(-0.180491107002967,0.00310177792423096,
0.00849425748487474));
#24893=CARTESIAN_POINT('Ctrl Pts',(-0.18,0.00310463170987884,0.00848584310919716));
#24894=CARTESIAN_POINT('Ctrl Pts',(-0.18,0.00333394220740964,0.00804665380354745));
#24895=CARTESIAN_POINT('Ctrl Pts',(-0.180492715511507,0.00208357847138839,
0.00778381458262853));
#24896=CARTESIAN_POINT('Ctrl Pts',(-0.18,0.00208768551873161,0.00777792629190908));
#24897=CARTESIAN_POINT('Ctrl Pts',(-0.18,0.00236958913814357,0.00737375990977421));
#24898=CARTESIAN_POINT('',(-0.180000000092441,0.002369415201346,0.00737400928367846));
#24899=CARTESIAN_POINT('',(-0.180492713748997,0.00208357848608163,0.00778381456156277));
#24900=CARTESIAN_POINT('Ctrl Pts',(-0.180000000092441,0.002369415201346,
0.00737400928367846));
#24901=CARTESIAN_POINT('Ctrl Pts',(-0.180000299553135,0.00208768401511753,
0.0077779284476468));
#24902=CARTESIAN_POINT('Ctrl Pts',(-0.180492713748996,0.00208357848608164,
0.00778381456156275));
#24903=CARTESIAN_POINT('',(-0.180000000073866,0.00163303568495152,0.0068004616007287));
#24904=CARTESIAN_POINT('Ctrl Pts',(-0.180000000073866,0.00163303568495152,
0.0068004616007287));
#24905=CARTESIAN_POINT('Ctrl Pts',(-0.180000000059821,0.00118804839875416,
0.00641493294655719));
#24906=CARTESIAN_POINT('Ctrl Pts',(-0.18,0.000780603533896183,0.00598502981387675));
#24907=CARTESIAN_POINT('Ctrl Pts',(-0.18,0.000418942701838473,0.00551967293650249));
#24908=CARTESIAN_POINT('Ctrl Pts',(-0.18,0.000249927081888821,0.0053021968535113));
#24909=CARTESIAN_POINT('Ctrl Pts',(-0.18,9.09590595398255E-5,0.00507695666847608));
#24910=CARTESIAN_POINT('Ctrl Pts',(-0.18,-5.70670721416072E-5,0.00484493104806877));
#24911=CARTESIAN_POINT('Ctrl Pts',(-0.18,-6.74294721945815E-5,0.00482868835987657));
#24912=CARTESIAN_POINT('Ctrl Pts',(-0.18,-7.77382685084171E-5,0.00481241242995712));
#24913=CARTESIAN_POINT('Ctrl Pts',(-0.18,-8.79933143911442E-5,0.00479610367742078));
#24914=CARTESIAN_POINT('Ctrl Pts',(-0.18,-0.000244740945435163,0.00454682558012237));
#24915=CARTESIAN_POINT('Ctrl Pts',(-0.179999999906675,-0.000388909840019564,
0.00428990581472337));
#24916=CARTESIAN_POINT('Ctrl Pts',(-0.180000000093167,-0.00052030903126298,
0.00402694496455378));
#24917=CARTESIAN_POINT('Ctrl Pts',(-0.180000000279659,-0.000651708222506395,
0.00376398411438418));
#24918=CARTESIAN_POINT('Ctrl Pts',(-0.18000000050776,-0.000769903124688603,
0.00349473306770954));
#24919=CARTESIAN_POINT('Ctrl Pts',(-0.180000000457489,-0.000874579938457122,
0.00322047030539096));
#24920=CARTESIAN_POINT('Ctrl Pts',(-0.180000000360256,-0.00107704602882691,
0.00268999075388821));
#24921=CARTESIAN_POINT('Ctrl Pts',(-0.180000000153618,-0.00122935539601011,
0.00214080127837629));
#24922=CARTESIAN_POINT('Ctrl Pts',(-0.180000000091491,-0.00132854406997328,
0.00158224127209026));
#24923=CARTESIAN_POINT('Ctrl Pts',(-0.180000000057257,-0.00138319974100772,
0.00127445943837102));
#24924=CARTESIAN_POINT('Ctrl Pts',(-0.18000000004624,-0.00142172317863241,
0.000963827247457888));
#24925=CARTESIAN_POINT('Ctrl Pts',(-0.180000000066894,-0.00144417813514861,
0.000651961194282699));
#24926=CARTESIAN_POINT('Ctrl Pts',(-0.180000000123781,-0.00150602452449947,
-0.000206993457269628));
#24927=CARTESIAN_POINT('Ctrl Pts',(-0.180000000048164,-0.00144517176436833,
-0.0010756726768805));
#24928=CARTESIAN_POINT('Ctrl Pts',(-0.180000000134111,-0.0012623500650625,
-0.00191796030930795));
#24929=CARTESIAN_POINT('Ctrl Pts',(-0.180000000165279,-0.00119605058425185,
-0.00222341219458856));
#24930=CARTESIAN_POINT('Ctrl Pts',(-0.180000000216682,-0.00111371887405417,
-0.00252539704694802));
#24931=CARTESIAN_POINT('Ctrl Pts',(-0.180000000371265,-0.00101602267705604,
-0.00282231615756755));
#24932=CARTESIAN_POINT('Ctrl Pts',(-0.180000000516477,-0.000924248987460435,
-0.00310123553345199));
#24933=CARTESIAN_POINT('Ctrl Pts',(-0.180000000323103,-0.0008186164521681,
-0.00337562307708563));
#24934=CARTESIAN_POINT('Ctrl Pts',(-0.180000000193685,-0.000699874970982025,
-0.00364426841946957));
#24935=CARTESIAN_POINT('Ctrl Pts',(-0.17999999994348,-0.000470313038758882,
-0.00416363825774677));
#24936=CARTESIAN_POINT('Ctrl Pts',(-0.180000000003078,-0.000191886024868714,
-0.0046617027692084));
#24937=CARTESIAN_POINT('Ctrl Pts',(-0.180000000003089,0.00013159832191248,
-0.00512867861339497));
#24938=CARTESIAN_POINT('Ctrl Pts',(-0.180000000003096,0.000310083227245415,
-0.00538633602455492));
#24939=CARTESIAN_POINT('Ctrl Pts',(-0.180000000005194,0.000502280903413068,
-0.00563452896521551));
#24940=CARTESIAN_POINT('Ctrl Pts',(-0.180000000017907,0.000706915973500765,
-0.00587200864424154));
#24941=CARTESIAN_POINT('Ctrl Pts',(-0.180000000029826,0.000898753882513541,
-0.00609463717530347));
#24942=CARTESIAN_POINT('Ctrl Pts',(-0.180000000008953,0.00110165204133482,
-0.00630779073382734));
#24943=CARTESIAN_POINT('Ctrl Pts',(-0.180000000005369,0.00131446604763071,
-0.00651061213963826));
#24944=CARTESIAN_POINT('Ctrl Pts',(-0.179999999998451,0.00172518580215862,
-0.00690204670476666));
#24945=CARTESIAN_POINT('Ctrl Pts',(-0.179999999991229,0.00217302812516551,
-0.00725489163512563));
#24946=CARTESIAN_POINT('Ctrl Pts',(-0.180000000010711,0.00265021480579363,
-0.00756184956024018));
#24947=CARTESIAN_POINT('Ctrl Pts',(-0.180000000021513,0.00291478944637761,
-0.00773204140759998));
#24948=CARTESIAN_POINT('Ctrl Pts',(-0.180000000040581,0.00318838199463977,
-0.00788813229953453));
#24949=CARTESIAN_POINT('Ctrl Pts',(-0.180000000141286,0.00346927698327818,
-0.00802948180824356));
#24950=CARTESIAN_POINT('Ctrl Pts',(-0.180000000235397,0.00373178266338216,
-0.0081615776106496));
#24951=CARTESIAN_POINT('Ctrl Pts',(-0.180000000150774,0.00400081715481969,
-0.00828058078675498));
#24952=CARTESIAN_POINT('Ctrl Pts',(-0.18000000009043,0.00427498444480135,
-0.00838619566190851));
#24953=CARTESIAN_POINT('Ctrl Pts',(-0.179999999973844,0.00480469075812819,
-0.00859024942103415));
#24954=CARTESIAN_POINT('Ctrl Pts',(-0.17999999998725,0.00535362645522928,
-0.00874446366426804));
#24955=CARTESIAN_POINT('Ctrl Pts',(-0.180000000024732,0.00591191863550963,
-0.00884508332764294));
#24956=CARTESIAN_POINT('Ctrl Pts',(-0.18000000004545,0.00622051505123686,
-0.00890070092102134));
#24957=CARTESIAN_POINT('Ctrl Pts',(-0.180000000083345,0.00653197023768919,
-0.00893994792029853));
#24958=CARTESIAN_POINT('Ctrl Pts',(-0.180000000289389,0.00684450224324547,
-0.00896290263578175));
#24959=CARTESIAN_POINT('Ctrl Pts',(-0.180000000482325,0.00713715030794149,
-0.00898439692418225));
#24960=CARTESIAN_POINT('Ctrl Pts',(-0.180000000600894,0.00743078154821022,
-0.00899143359818871));
#24961=CARTESIAN_POINT('Ctrl Pts',(-0.18000000053753,0.00772406620072347,
-0.0089840730882348));
#24962=CARTESIAN_POINT('Ctrl Pts',(-0.180000000414596,0.00829307322193137,
-0.00896979282567229));
#24963=CARTESIAN_POINT('Ctrl Pts',(-0.180000000392808,0.00886085876197087,
-0.00890178007901912));
#24964=CARTESIAN_POINT('Ctrl Pts',(-0.180000000358353,0.00941741794215845,
-0.00877991725364757));
#24965=CARTESIAN_POINT('Ctrl Pts',(-0.180000000339531,0.00972146465792907,
-0.00871334393467678));
#24966=CARTESIAN_POINT('Ctrl Pts',(-0.180000000318419,0.0100221583669829,
-0.00863069319347393));
#24967=CARTESIAN_POINT('Ctrl Pts',(-0.180000000285255,0.0103179911779754,
-0.00853255598738525));
#24968=CARTESIAN_POINT('Ctrl Pts',(-0.180000000222673,0.0108762287736087,
-0.00834737072079723));
#24969=CARTESIAN_POINT('Ctrl Pts',(-0.18,0.0114171707809986,-0.00810658998512941));
#24970=CARTESIAN_POINT('Ctrl Pts',(-0.18,0.0119298368797898,-0.00781556806782665));
#24971=CARTESIAN_POINT('Ctrl Pts',(-0.18,0.0121696484903194,-0.0076794357297369));
#24972=CARTESIAN_POINT('Ctrl Pts',(-0.18,0.0124032195712773,-0.00753222783046099));
#24973=CARTESIAN_POINT('Ctrl Pts',(-0.18,0.0126293472179787,-0.0073745016803242));
#24974=CARTESIAN_POINT('Ctrl Pts',(-0.18,0.0126449259219565,-0.00736363538848248));
#24975=CARTESIAN_POINT('Ctrl Pts',(-0.18,0.0126604693095513,-0.00735271919189223));
#24976=CARTESIAN_POINT('Ctrl Pts',(-0.18,0.0126759770760497,-0.00734175340323608));
#24977=CARTESIAN_POINT('Ctrl Pts',(-0.18,0.0129165828191756,-0.00717161725056425));
#24978=CARTESIAN_POINT('Ctrl Pts',(-0.179999999946229,0.0131485905079609,
-0.00698955702291025));
#24979=CARTESIAN_POINT('Ctrl Pts',(-0.180000000053711,0.0133711230714489,
-0.00679686694357883));
#24980=CARTESIAN_POINT('Ctrl Pts',(-0.180000000161193,0.013593655634937,
-0.00660417686424741));
#24981=CARTESIAN_POINT('Ctrl Pts',(-0.18000000018702,0.0138064196112521,
-0.00640048280567611));
#24982=CARTESIAN_POINT('Ctrl Pts',(-0.180000000112277,0.0140085963705019,
-0.00618691252231924));
#24983=CARTESIAN_POINT('Ctrl Pts',(-0.179999999967716,0.0143996253669064,
-0.00577384737144471));
#24984=CARTESIAN_POINT('Ctrl Pts',(-0.179999999997186,0.0147514853889812,
-0.00532407927780652));
#24985=CARTESIAN_POINT('Ctrl Pts',(-0.180000000012131,0.0150570930156507,
-0.00484509518207374));
#24986=CARTESIAN_POINT('Ctrl Pts',(-0.180000000020367,0.0152255174438687,
-0.00458112067551943));
#24987=CARTESIAN_POINT('Ctrl Pts',(-0.180000000036385,0.0153798945654668,
-0.00430827187588287));
#24988=CARTESIAN_POINT('Ctrl Pts',(-0.18000000012645,0.0155196673863458,
-0.00402817957933301));
#24989=CARTESIAN_POINT('Ctrl Pts',(-0.180000000210945,0.0156507980032042,
-0.00376540549068789));
#24990=CARTESIAN_POINT('Ctrl Pts',(-0.180000000145609,0.0157688706720626,
-0.00349613328218849));
#24991=CARTESIAN_POINT('Ctrl Pts',(-0.180000000087433,0.0158735896851957,
-0.00322174217319132));
#24992=CARTESIAN_POINT('Ctrl Pts',(-0.179999999974608,0.0160766802466698,
-0.00268959196739333));
#24993=CARTESIAN_POINT('Ctrl Pts',(-0.179999999994891,0.0162297495161568,
-0.00213813714056621));
#24994=CARTESIAN_POINT('Ctrl Pts',(-0.180000000013797,0.0163292338388839,
-0.00157729922827135));
#24995=CARTESIAN_POINT('Ctrl Pts',(-0.180000000024137,0.0163836399779672,
-0.00127058733012421));
#24996=CARTESIAN_POINT('Ctrl Pts',(-0.180000000043723,0.0164220223554685,
-0.000961069827483446));
#24997=CARTESIAN_POINT('Ctrl Pts',(-0.180000000149483,0.016444429808688,
-0.000650446720184491));
#24998=CARTESIAN_POINT('Ctrl Pts',(-0.180000000443122,0.0165066437688952,
0.000211993711915339));
#24999=CARTESIAN_POINT('Ctrl Pts',(-0.180000000296702,0.0164447645933107,
0.00108345095688852));
#25000=CARTESIAN_POINT('Ctrl Pts',(-0.180000000268535,0.0162603541706888,
0.0019278501776853));
#25001=CARTESIAN_POINT('Ctrl Pts',(-0.180000000258442,0.016194273293351,
0.0022304287442339));
#25002=CARTESIAN_POINT('Ctrl Pts',(-0.180000000268355,0.016112459702564,
0.00252954106943733));
#25003=CARTESIAN_POINT('Ctrl Pts',(-0.18000000035993,0.0160155755183459,
0.00282367481902353));
#25004=CARTESIAN_POINT('Ctrl Pts',(-0.180000000446714,0.0159237613421876,
0.00310241637128562));
#25005=CARTESIAN_POINT('Ctrl Pts',(-0.180000000236453,0.0158181267106129,
0.00337660925175313));
#25006=CARTESIAN_POINT('Ctrl Pts',(-0.180000000141743,0.0156994560460536,
0.00364506614002243));
#25007=CARTESIAN_POINT('Ctrl Pts',(-0.179999999957256,0.0154682929609363,
0.00416800348720764));
#25008=CARTESIAN_POINT('Ctrl Pts',(-0.180000000001891,0.0151875969475736,
0.00466925202736088));
#25009=CARTESIAN_POINT('Ctrl Pts',(-0.180000000003811,0.0148613567562351,
0.00513883810306275));
#25010=CARTESIAN_POINT('Ctrl Pts',(-0.180000000004847,0.0146851576377794,
0.00539245692371836));
#25011=CARTESIAN_POINT('Ctrl Pts',(-0.180000000008273,0.0144956778303638,
0.005636840304416));
#25012=CARTESIAN_POINT('Ctrl Pts',(-0.180000000027596,0.014294151952822,
0.00587080597888225));
#25013=CARTESIAN_POINT('Ctrl Pts',(-0.180000000045963,0.014102598737904,
0.00609319368249218));
#25014=CARTESIAN_POINT('Ctrl Pts',(-0.180000000030252,0.0139000517862225,
0.00630612585062232));
#25015=CARTESIAN_POINT('Ctrl Pts',(-0.18000000001814,0.0136875780978067,
0.00650871390624616));
#25016=CARTESIAN_POINT('Ctrl Pts',(-0.179999999994542,0.0132736146987159,
0.00690341708453866));
#25017=CARTESIAN_POINT('Ctrl Pts',(-0.179999999993531,0.0128219471861013,
0.00725894839754447));
#25018=CARTESIAN_POINT('Ctrl Pts',(-0.180000000009742,0.0123403444657045,
0.00756790445316537));
#25019=CARTESIAN_POINT('Ctrl Pts',(-0.180000000018493,0.0120803750574165,
0.00773467909866692));
#25020=CARTESIAN_POINT('Ctrl Pts',(-0.180000000034388,0.0118116845160434,
0.00788788425791664));
#25021=CARTESIAN_POINT('Ctrl Pts',(-0.180000000114831,0.0115358336793546,
0.00802690888367712));
#25022=CARTESIAN_POINT('Ctrl Pts',(-0.180000000191321,0.0112735421870466,
0.00815909980611903));
#25023=CARTESIAN_POINT('Ctrl Pts',(-0.180000000129546,0.0110046518767973,
0.00827827701382785));
#25024=CARTESIAN_POINT('Ctrl Pts',(-0.180000000077698,0.0107305462975331,
0.00838407719408214));
#25025=CARTESIAN_POINT('Ctrl Pts',(-0.179999999976826,0.0101972512619832,
0.00858992017999054));
#25026=CARTESIAN_POINT('Ctrl Pts',(-0.179999999991605,0.0096441953899426,
0.00874529488330738));
#25027=CARTESIAN_POINT('Ctrl Pts',(-0.180000000019558,0.0090814082947659,
0.00884626362895226));
#25028=CARTESIAN_POINT('Ctrl Pts',(-0.180000000034707,0.00877640323489228,
0.00890098410597584));
#25029=CARTESIAN_POINT('Ctrl Pts',(-0.180000000063481,0.00846854136355709,
0.00893972891457769));
#25030=CARTESIAN_POINT('Ctrl Pts',(-0.180000000199897,0.00815953756376133,
0.00896253601849186));
#25031=CARTESIAN_POINT('Ctrl Pts',(-0.180000000329273,0.00786648114315136,
0.00898416607042646));
#25032=CARTESIAN_POINT('Ctrl Pts',(-0.180000000237125,0.00757234589332953,
0.00899118671439754));
#25033=CARTESIAN_POINT('Ctrl Pts',(-0.180000000142269,0.00727854544340191,
0.00898381724086646));
#25034=CARTESIAN_POINT('Ctrl Pts',(-0.179999999957967,0.00670769761841669,
0.00896949851556314));
#25035=CARTESIAN_POINT('Ctrl Pts',(-0.179999999987481,0.0061380290887039,
0.00890113003428405));
#25036=CARTESIAN_POINT('Ctrl Pts',(-0.180000000028244,0.00558017359327183,
0.00877894937833312));
#25037=CARTESIAN_POINT('Ctrl Pts',(-0.18000000005042,0.0052766881758777,
0.00871248046716817));
#25038=CARTESIAN_POINT('Ctrl Pts',(-0.180000000091846,0.00497669798505343,
0.00863008892616214));
#25039=CARTESIAN_POINT('Ctrl Pts',(-0.180000000311714,0.0046817845363248,
0.00853248488801863));
#25040=CARTESIAN_POINT('Ctrl Pts',(-0.180000000519721,0.00440278044521801,
0.00844014618299184));
#25041=CARTESIAN_POINT('Ctrl Pts',(-0.180000000511612,0.00412836853147088,
0.00833392835474274));
#25042=CARTESIAN_POINT('Ctrl Pts',(-0.180000000373709,0.00385978342259457,
0.00821449183257972));
#25043=CARTESIAN_POINT('Ctrl Pts',(-0.180000000105832,0.00333805554982461,
0.00798248581072742));
#25044=CARTESIAN_POINT('Ctrl Pts',(-0.18000000010862,0.00283804754615616,
0.00770103805887969));
#25045=CARTESIAN_POINT('Ctrl Pts',(-0.180000000092441,0.002369415201346,
0.00737400928367846));
#25046=CARTESIAN_POINT('',(-0.180494077221453,0.00130607217168702,0.00717829214732416));
#25047=CARTESIAN_POINT('Ctrl Pts',(-0.180000000073866,0.00163303568495152,
0.0068004616007287));
#25048=CARTESIAN_POINT('Ctrl Pts',(-0.180000268510106,0.00130973850057992,
0.00717346067102031));
#25049=CARTESIAN_POINT('Ctrl Pts',(-0.180494077221453,0.00130607217168702,
0.00717829214732417));
#25050=CARTESIAN_POINT('',(-0.180505050469422,0.0166467264643195,0.00245334977916771));
#25051=CARTESIAN_POINT('Ctrl Pts',(-0.180505050469422,0.0166467264643195,
0.0024533497791677));
#25052=CARTESIAN_POINT('Ctrl Pts',(-0.180505306133657,0.0166837724953881,
0.00231446224061256));
#25053=CARTESIAN_POINT('Ctrl Pts',(-0.180505550682239,0.0167176593319398,
0.00217472825564444));
#25054=CARTESIAN_POINT('Ctrl Pts',(-0.180505778846172,0.0167483294518472,
0.00203428715171698));
#25055=CARTESIAN_POINT('Ctrl Pts',(-0.180507226251443,0.016942891723494,
0.00114336985842741));
#25056=CARTESIAN_POINT('Ctrl Pts',(-0.180508014307505,0.0170079758680575,
0.000223993120464905));
#25057=CARTESIAN_POINT('Ctrl Pts',(-0.18050756952682,0.0169427469804377,
-0.000685980192934213));
#25058=CARTESIAN_POINT('Ctrl Pts',(-0.180507409214296,0.0169192364999648,
-0.00101396232778566));
#25059=CARTESIAN_POINT('Ctrl Pts',(-0.180507095715993,0.0168787986842539,
-0.00134074577739527));
#25060=CARTESIAN_POINT('Ctrl Pts',(-0.180506641320586,0.0168213956365477,
-0.00166456445752732));
#25061=CARTESIAN_POINT('Ctrl Pts',(-0.180505382372451,0.016662354724553,
-0.00256173665076423));
#25062=CARTESIAN_POINT('Ctrl Pts',(-0.180503042799424,0.016373071623164,
-0.00343614135643362));
#25063=CARTESIAN_POINT('Ctrl Pts',(-0.180501039464594,0.0159665378030119,
-0.00425159980508381));
#25064=CARTESIAN_POINT('Ctrl Pts',(-0.18050031302138,0.0158191217393433,
-0.00454729888010876));
#25065=CARTESIAN_POINT('Ctrl Pts',(-0.180499580110058,0.0156562625227054,
-0.00483530720101641));
#25066=CARTESIAN_POINT('Ctrl Pts',(-0.180498891082393,0.0154785401533995,
-0.00511392775516268));
#25067=CARTESIAN_POINT('Ctrl Pts',(-0.180496994130169,0.0149892552365115,
-0.00588099402381038));
#25068=CARTESIAN_POINT('Ctrl Pts',(-0.180495429923449,0.0143873379575043,
-0.00657696679982974));
#25069=CARTESIAN_POINT('Ctrl Pts',(-0.180494085708543,0.0136985260558778,
-0.00717437305409498));
#25070=CARTESIAN_POINT('Ctrl Pts',(-0.180493597855415,0.0134485369807919,
-0.0073911884671296));
#25071=CARTESIAN_POINT('Ctrl Pts',(-0.180493140703323,0.0131869995586514,
-0.0075950898795007));
#25072=CARTESIAN_POINT('Ctrl Pts',(-0.180492709092622,0.0129152983549508,
-0.0077845977543531));
#25073=CARTESIAN_POINT('Ctrl Pts',(-0.180491519488495,0.0121664363094803,
-0.00830691879254459));
#25074=CARTESIAN_POINT('Ctrl Pts',(-0.180490524505021,0.0113402538840803,
-0.00871961155206156));
#25075=CARTESIAN_POINT('Ctrl Pts',(-0.180489841473695,0.010475431349535,
-0.00900643654204879));
#25076=CARTESIAN_POINT('Ctrl Pts',(-0.18048959464343,0.0101629063354497,
-0.00911008784674441));
#25077=CARTESIAN_POINT('Ctrl Pts',(-0.180489384500336,0.00984527055527501,
-0.00919737486172379));
#25078=CARTESIAN_POINT('Ctrl Pts',(-0.180489215197301,0.00952409565645105,
-0.00926767275065503));
#25079=CARTESIAN_POINT('Ctrl Pts',(-0.18048874602362,0.00863405367343233,
-0.00946248272084727));
#25080=CARTESIAN_POINT('Ctrl Pts',(-0.180488590053928,0.00771686160166094,
-0.00952699527599385));
#25081=CARTESIAN_POINT('Ctrl Pts',(-0.180488753127145,0.0068087871965689,
-0.00946093879366742));
#25082=CARTESIAN_POINT('Ctrl Pts',(-0.18048881243083,0.00647855419143593,
-0.00943691649929942));
#25083=CARTESIAN_POINT('Ctrl Pts',(-0.180488913882774,0.00614947823465072,
-0.00939559647679476));
#25084=CARTESIAN_POINT('Ctrl Pts',(-0.180489057263567,0.00582343159064595,
-0.0093369096156809));
#25085=CARTESIAN_POINT('Ctrl Pts',(-0.180489450424322,0.00492938753887127,
-0.00917598589491597));
#25086=CARTESIAN_POINT('Ctrl Pts',(-0.180490159006754,0.00405811752998488,
-0.00888442947496311));
#25087=CARTESIAN_POINT('Ctrl Pts',(-0.180491091913702,0.0032456634858749,
-0.00847615964082623));
#25088=CARTESIAN_POINT('Ctrl Pts',(-0.180491432870738,0.00294872934590647,
-0.00832694596781499));
#25089=CARTESIAN_POINT('Ctrl Pts',(-0.180491810468584,0.00265955199509477,
-0.00816209795373336));
#25090=CARTESIAN_POINT('Ctrl Pts',(-0.180492218351403,0.00237992845554504,
-0.00798230320031856));
#25091=CARTESIAN_POINT('Ctrl Pts',(-0.180493333494458,0.00161544357674557,
-0.00749074812418146));
#25092=CARTESIAN_POINT('Ctrl Pts',(-0.180494675200404,0.000922426457022649,
-0.00688739759659587));
#25093=CARTESIAN_POINT('Ctrl Pts',(-0.180496337220057,0.000329090474573647,
-0.00619926450814251));
#25094=CARTESIAN_POINT('Ctrl Pts',(-0.180496943504142,0.000112648892505816,
-0.00594824212159634));
#25095=CARTESIAN_POINT('Ctrl Pts',(-0.180497578128166,-9.05934709865707E-5,
-0.00568588146362153));
#25096=CARTESIAN_POINT('Ctrl Pts',(-0.180498255087495,-0.000279289301226472,
-0.005413481592156));
#25097=CARTESIAN_POINT('Ctrl Pts',(-0.180500112668822,-0.000797072033236919,
-0.00466601436160086));
#25098=CARTESIAN_POINT('Ctrl Pts',(-0.180502288445076,-0.00120528133270418,
-0.00384294365333793));
#25099=CARTESIAN_POINT('Ctrl Pts',(-0.180504030056536,-0.00148980242281501,
-0.0029799515977759));
#25100=CARTESIAN_POINT('Ctrl Pts',(-0.180504663447986,-0.00159327741133636,
-0.00266609755972017));
#25101=CARTESIAN_POINT('Ctrl Pts',(-0.180505273972546,-0.00168044127198726,
-0.00234683231956376));
#25102=CARTESIAN_POINT('Ctrl Pts',(-0.180505797177316,-0.00175059117883485,
-0.00202388931840672));
#25103=CARTESIAN_POINT('Ctrl Pts',(-0.180507236890724,-0.00194362413133551,
-0.00113524036926128));
#25104=CARTESIAN_POINT('Ctrl Pts',(-0.180508014788672,-0.00200773829548467,
-0.000218750017278828));
#25105=CARTESIAN_POINT('Ctrl Pts',(-0.18050756675746,-0.00194262103711012,
0.000687516385167797));
#25106=CARTESIAN_POINT('Ctrl Pts',(-0.18050740395279,-0.00191895886023441,
0.00101683362680998));
#25107=CARTESIAN_POINT('Ctrl Pts',(-0.180507087365724,-0.0018782492411139,
0.00134480018749305));
#25108=CARTESIAN_POINT('Ctrl Pts',(-0.18050662968436,-0.0018204757856677,
0.00166974486293542));
#25109=CARTESIAN_POINT('Ctrl Pts',(-0.180505370126551,-0.0016614808760678,
0.00256400588467813));
#25110=CARTESIAN_POINT('Ctrl Pts',(-0.180503042831105,-0.00137339807730806,
0.00343545636344477));
#25111=CARTESIAN_POINT('Ctrl Pts',(-0.180501042736115,-0.000967262940565802,
0.00425032043965544));
#25112=CARTESIAN_POINT('Ctrl Pts',(-0.180500316492093,-0.000819793337187815,
0.0045462014685407));
#25113=CARTESIAN_POINT('Ctrl Pts',(-0.180499582732681,-0.000656707144888704,
0.00483465770437334));
#25114=CARTESIAN_POINT('Ctrl Pts',(-0.180498892503896,-0.000478610824537603,
0.00511381696861555));
#25115=CARTESIAN_POINT('Ctrl Pts',(-0.180496991097895,1.19995639816014E-5,
0.00588283024647891));
#25116=CARTESIAN_POINT('Ctrl Pts',(-0.180495421036052,0.000616709580096667,
0.00658110736474186));
#25117=CARTESIAN_POINT('Ctrl Pts',(-0.180494077221384,0.00130607220731985,
0.00717829217819236));
#25118=CARTESIAN_POINT('Ctrl Pts',(-0.180492713748997,0.00208357848608163,
0.00778381456156277));
#25119=CARTESIAN_POINT('Ctrl Pts',(-0.180491527231616,0.00283280398077721,
0.00830658235132092));
#25120=CARTESIAN_POINT('Ctrl Pts',(-0.180490539611414,0.00365797125397222,
0.00871895924666266));
#25121=CARTESIAN_POINT('Ctrl Pts',(-0.180489844972134,0.00452428905665735,
0.0090063203212091));
#25122=CARTESIAN_POINT('Ctrl Pts',(-0.180489595209188,0.00483578034829864,
0.00910964322649913));
#25123=CARTESIAN_POINT('Ctrl Pts',(-0.180489383382281,0.00515266432219857,
0.00919681506862515));
#25124=CARTESIAN_POINT('Ctrl Pts',(-0.180489213232927,0.00547326492548861,
0.00926709504263265));
#25125=CARTESIAN_POINT('Ctrl Pts',(-0.180488740001119,0.00636494273336552,
0.00946256283813135));
#25126=CARTESIAN_POINT('Ctrl Pts',(-0.180488589317135,0.00728538046776418,
0.00952730360716332));
#25127=CARTESIAN_POINT('Ctrl Pts',(-0.180488753931549,0.00819563487316819,
0.00946063692069833));
#25128=CARTESIAN_POINT('Ctrl Pts',(-0.18048881296935,0.00852209120843912,
0.00943672738286055));
#25129=CARTESIAN_POINT('Ctrl Pts',(-0.180488913061566,0.00884732386434948,
0.00939591666247467));
#25130=CARTESIAN_POINT('Ctrl Pts',(-0.180489054012028,0.00916952818551784,
0.00933817345182018));
#25131=CARTESIAN_POINT('Ctrl Pts',(-0.180489447378089,0.0100687394631446,
0.00917702307978729));
#25132=CARTESIAN_POINT('Ctrl Pts',(-0.180490159114969,0.0109443343949455,
0.00888392857305358));
#25133=CARTESIAN_POINT('Ctrl Pts',(-0.180491097780424,0.0117599091286999,
0.00847339840641515));
#25134=CARTESIAN_POINT('Ctrl Pts',(-0.180491433329071,0.0120514560236885,
0.00832664447887299));
#25135=CARTESIAN_POINT('Ctrl Pts',(-0.180491803878337,0.0123354002447643,
0.00816486104868504));
#25136=CARTESIAN_POINT('Ctrl Pts',(-0.1804922034718,0.0126101076158722,
0.00798869938687643));
#25137=CARTESIAN_POINT('Ctrl Pts',(-0.180493322240716,0.0133792244714115,
0.00749548763631303));
#25138=CARTESIAN_POINT('Ctrl Pts',(-0.180494668822925,0.0140759154697159,
0.00688956279261156));
#25139=CARTESIAN_POINT('Ctrl Pts',(-0.180496341168924,0.0146721295242753,
0.00619783709289612));
#25140=CARTESIAN_POINT('Ctrl Pts',(-0.180496938961584,0.0148852507239376,
0.00595057453705201));
#25141=CARTESIAN_POINT('Ctrl Pts',(-0.180497564189998,0.0150855886906841,
0.00569228752533243));
#25142=CARTESIAN_POINT('Ctrl Pts',(-0.180498230460235,0.0152718433472023,
0.00542420786392051));
#25143=CARTESIAN_POINT('Ctrl Pts',(-0.180500093843356,0.0157927487763465,
0.0046744593546316));
#25144=CARTESIAN_POINT('Ctrl Pts',(-0.180502277572748,0.0162034481788898,
0.00384810331139103));
#25145=CARTESIAN_POINT('Ctrl Pts',(-0.180504027062762,0.0164893813621227,
0.0029812596211392));
#25146=CARTESIAN_POINT('Ctrl Pts',(-0.180504379031403,0.0165469064197915,
0.00280686491567759));
#25147=CARTESIAN_POINT('Ctrl Pts',(-0.180504723822302,0.0165993949346352,
0.00263079819845253));
#25148=CARTESIAN_POINT('Ctrl Pts',(-0.180505050469422,0.0166467264643195,
0.0024533497791677));
#25149=CARTESIAN_POINT('Ctrl Pts',(-0.238376419148325,0.0160572510994551,
0.00229523935965256));
#25150=CARTESIAN_POINT('Ctrl Pts',(-0.180143329927774,0.0166506887410553,
0.00245441214111993));
#25151=CARTESIAN_POINT('Ctrl Pts',(-0.238376419148325,0.0160499153270237,
0.00339695540894448));
#25152=CARTESIAN_POINT('Ctrl Pts',(-0.180143329927774,0.0163802403000704,
0.00346535234146251));
#25153=CARTESIAN_POINT('Ctrl Pts',(-0.238376419148325,0.0156043581343594,
0.00560766010208411));
#25154=CARTESIAN_POINT('Ctrl Pts',(-0.180143329927774,0.0155045639563625,
0.00538672371465897));
#25155=CARTESIAN_POINT('Ctrl Pts',(-0.238376419148325,0.0137116283891667,
0.00844195664423076));
#25156=CARTESIAN_POINT('Ctrl Pts',(-0.180143329927774,0.0133464539612027,
0.00767441593321455));
#25157=CARTESIAN_POINT('Ctrl Pts',(-0.238376419148325,0.0108665999736013,
0.0103474435450232));
#25158=CARTESIAN_POINT('Ctrl Pts',(-0.180143329927774,0.0105817751956803,
0.00914209790934899));
#25159=CARTESIAN_POINT('Ctrl Pts',(-0.238376419148325,0.0075,0.0110189940848823));
#25160=CARTESIAN_POINT('Ctrl Pts',(-0.180143329927774,0.0075,0.00964748427001006));
#25161=CARTESIAN_POINT('Ctrl Pts',(-0.238376419148325,0.00413340002639867,
0.0103474435450232));
#25162=CARTESIAN_POINT('Ctrl Pts',(-0.180143329927774,0.0044182248043197,
0.00914209790934899));
#25163=CARTESIAN_POINT('Ctrl Pts',(-0.238376419148325,0.00128837161083331,
0.00844195664423074));
#25164=CARTESIAN_POINT('Ctrl Pts',(-0.180143329927774,0.00165354603879735,
0.00767441593321453));
#25165=CARTESIAN_POINT('Ctrl Pts',(-0.238376419148325,-0.000604358134359394,
0.00560766010208411));
#25166=CARTESIAN_POINT('Ctrl Pts',(-0.180143329927774,-0.000504563956362522,
0.00538672371465897));
#25167=CARTESIAN_POINT('Ctrl Pts',(-0.238376419148325,-0.00104991532702373,
0.00339695540894447));
#25168=CARTESIAN_POINT('Ctrl Pts',(-0.180143329927774,-0.00138024030007043,
0.00346535234146251));
#25169=CARTESIAN_POINT('Ctrl Pts',(-0.238376419148325,-0.00105996989569538,
0.00188691951593846));
#25170=CARTESIAN_POINT('Ctrl Pts',(-0.180143329927774,-0.00175092279430951,
0.00207973579427586));
#25171=CARTESIAN_POINT('Ctrl Pts',(-0.238376419148325,-0.00106440179407383,
0.00111305841215638));
#25172=CARTESIAN_POINT('Ctrl Pts',(-0.180143329927774,-0.00191431390523475,
0.0012839986244053));
#25173=CARTESIAN_POINT('Ctrl Pts',(-0.238376419148325,-0.00106680965804379,
-1.88715094039015E-18));
#25174=CARTESIAN_POINT('Ctrl Pts',(-0.180143329927774,-0.00200308479649061,
-3.46556198647675E-18));
#25175=CARTESIAN_POINT('Ctrl Pts',(-0.238376419148325,-0.00106440179407383,
-0.00111305841215639));
#25176=CARTESIAN_POINT('Ctrl Pts',(-0.180143329927774,-0.00191431390523475,
-0.0012839986244053));
#25177=CARTESIAN_POINT('Ctrl Pts',(-0.238376419148325,-0.00105996989569538,
-0.00188691951593846));
#25178=CARTESIAN_POINT('Ctrl Pts',(-0.180143329927774,-0.00175092279430951,
-0.00207973579427587));
#25179=CARTESIAN_POINT('Ctrl Pts',(-0.238376419148325,-0.00104991532702373,
-0.00339695540894448));
#25180=CARTESIAN_POINT('Ctrl Pts',(-0.180143329927774,-0.00138024030007042,
-0.00346535234146251));
#25181=CARTESIAN_POINT('Ctrl Pts',(-0.238376419148325,-0.000604358134359395,
-0.00560766010208411));
#25182=CARTESIAN_POINT('Ctrl Pts',(-0.180143329927774,-0.000504563956362519,
-0.00538672371465899));
#25183=CARTESIAN_POINT('Ctrl Pts',(-0.238376419148325,0.00128837161083331,
-0.00844195664423075));
#25184=CARTESIAN_POINT('Ctrl Pts',(-0.180143329927774,0.00165354603879737,
-0.00767441593321454));
#25185=CARTESIAN_POINT('Ctrl Pts',(-0.238376419148325,0.00413340002639866,
-0.0103474435450231));
#25186=CARTESIAN_POINT('Ctrl Pts',(-0.180143329927774,0.0044182248043197,
-0.00914209790934901));
#25187=CARTESIAN_POINT('Ctrl Pts',(-0.238376419148325,0.0075,-0.0110189940848823));
#25188=CARTESIAN_POINT('Ctrl Pts',(-0.180143329927774,0.0075,-0.00964748427001004));
#25189=CARTESIAN_POINT('Ctrl Pts',(-0.238376419148325,0.0108665999736013,
-0.0103474435450232));
#25190=CARTESIAN_POINT('Ctrl Pts',(-0.180143329927774,0.0105817751956803,
-0.00914209790934901));
#25191=CARTESIAN_POINT('Ctrl Pts',(-0.238376419148325,0.0137116283891667,
-0.00844195664423074));
#25192=CARTESIAN_POINT('Ctrl Pts',(-0.180143329927774,0.0133464539612027,
-0.00767441593321454));
#25193=CARTESIAN_POINT('Ctrl Pts',(-0.238376419148325,0.0156043581343594,
-0.00560766010208412));
#25194=CARTESIAN_POINT('Ctrl Pts',(-0.180143329927774,0.0155045639563625,
-0.00538672371465897));
#25195=CARTESIAN_POINT('Ctrl Pts',(-0.238376419148325,0.0160499153270237,
-0.00339695540894448));
#25196=CARTESIAN_POINT('Ctrl Pts',(-0.180143329927774,0.0163802403000704,
-0.00346535234146251));
#25197=CARTESIAN_POINT('Ctrl Pts',(-0.238376419148325,0.0160599698956954,
-0.00188691951593846));
#25198=CARTESIAN_POINT('Ctrl Pts',(-0.180143329927774,0.0167509227943095,
-0.00207973579427587));
#25199=CARTESIAN_POINT('Ctrl Pts',(-0.238376419148325,0.0160644017940738,
-0.00111305841215638));
#25200=CARTESIAN_POINT('Ctrl Pts',(-0.180143329927774,0.0169143139052348,
-0.0012839986244053));
#25201=CARTESIAN_POINT('Ctrl Pts',(-0.238376419148325,0.0160668096580438,
-5.5742513075403E-20));
#25202=CARTESIAN_POINT('Ctrl Pts',(-0.180143329927774,0.0170030847964906,
-2.05506317145176E-18));
#25203=CARTESIAN_POINT('Ctrl Pts',(-0.238376419148325,0.0160644017940738,
0.00111305841215638));
#25204=CARTESIAN_POINT('Ctrl Pts',(-0.180143329927774,0.0169143139052348,
0.0012839986244053));
#25205=CARTESIAN_POINT('Ctrl Pts',(-0.238376419148325,0.0160599698956954,
0.00188691951593846));
#25206=CARTESIAN_POINT('Ctrl Pts',(-0.180143329927774,0.0167509227943095,
0.00207973579427586));
#25207=CARTESIAN_POINT('Ctrl Pts',(-0.238376419148325,0.0160572510994551,
0.00229523935965256));
#25208=CARTESIAN_POINT('Ctrl Pts',(-0.180143329927774,0.0166506887410553,
0.00245441214111993));
#25209=CARTESIAN_POINT('',(-0.238020422914454,0.0160608789606638,0.00229621243031557));
#25210=CARTESIAN_POINT('Ctrl Pts',(-0.180505053483848,0.0166470025142571,
0.00245342341554633));
#25211=CARTESIAN_POINT('Ctrl Pts',(-0.238020422914454,0.0160608789606638,
0.00229621243031557));
#25212=CARTESIAN_POINT('',(-0.237977937649492,0.00102548423602744,0.00782605181637851));
#25213=CARTESIAN_POINT('Ctrl Pts',(-0.180494073660068,0.00130587316507919,
0.0071785219603984));
#25214=CARTESIAN_POINT('Ctrl Pts',(-0.237977933526904,0.00102520228666307,
0.00782629549301537));
#25215=CARTESIAN_POINT('',(-0.238020316532522,-0.00106075457250487,0.00231025307800846));
#25216=CARTESIAN_POINT('Ctrl Pts',(-0.238020318599055,-0.00106098169283407,
0.00231040371569406));
#25217=CARTESIAN_POINT('Ctrl Pts',(-0.238014604516959,-0.00105350020411119,
0.00306190054704093));
#25218=CARTESIAN_POINT('Ctrl Pts',(-0.238004107697475,-0.000841551378611133,
0.00446246739893098));
#25219=CARTESIAN_POINT('Ctrl Pts',(-0.237993318101237,-0.00027785053263636,
0.00587614678579025));
#25220=CARTESIAN_POINT('Ctrl Pts',(-0.237986081899084,0.000251531250557718,
0.00680176374543222));
#25221=CARTESIAN_POINT('Ctrl Pts',(-0.237981570675819,0.000647625364551933,
0.00737065558877918));
#25222=CARTESIAN_POINT('Ctrl Pts',(-0.237979022233705,0.000907805533526721,
0.00768990840376775));
#25223=CARTESIAN_POINT('Ctrl Pts',(-0.237977937649492,0.00102548423602743,
0.00782605181637851));
#25224=CARTESIAN_POINT('',(-0.238020316532533,-0.00106075457252077,-0.0023102530755598));
#25225=CARTESIAN_POINT('Ctrl Pts',(-0.238020316619813,-0.00106075405523068,
-0.00231028189603671));
#25226=CARTESIAN_POINT('Ctrl Pts',(-0.238020352159604,-0.00106079956504005,
-0.00230559487996849));
#25227=CARTESIAN_POINT('Ctrl Pts',(-0.238020387591151,-0.00106084120528452,
-0.00230090505001212));
#25228=CARTESIAN_POINT('Ctrl Pts',(-0.238020422914453,-0.0010608789606638,
-0.00229621243031556));
#25229=CARTESIAN_POINT('Ctrl Pts',(-0.238023371086054,-0.0010640301194925,
-0.00190455459856342));
#25230=CARTESIAN_POINT('Ctrl Pts',(-0.238025565230501,-0.00106677025071908,
-0.00151323660125846));
#25231=CARTESIAN_POINT('Ctrl Pts',(-0.238027005347795,-0.00106864274316786,
-0.00112190150667839));
#25232=CARTESIAN_POINT('Ctrl Pts',(-0.238028380588602,-0.00107043088086772,
-0.000748195841613378));
#25233=CARTESIAN_POINT('Ctrl Pts',(-0.238029068209006,-0.0010714200523582,
-0.000374041179707509));
#25234=CARTESIAN_POINT('Ctrl Pts',(-0.238029068209006,-0.0010714200523582,
-5.10251228893053E-18));
#25235=CARTESIAN_POINT('Ctrl Pts',(-0.238029068209005,-0.0010714200523582,
0.000374041179701486));
#25236=CARTESIAN_POINT('Ctrl Pts',(-0.238028380588602,-0.00107043088086775,
0.000748195841607102));
#25237=CARTESIAN_POINT('Ctrl Pts',(-0.238027005347795,-0.00106864274316786,
0.00112190150667838));
#25238=CARTESIAN_POINT('Ctrl Pts',(-0.238025565230501,-0.00106677025071912,
0.00151323660125024));
#25239=CARTESIAN_POINT('Ctrl Pts',(-0.238023371086054,-0.00106403011949258,
0.00190455459855405));
#25240=CARTESIAN_POINT('Ctrl Pts',(-0.238020422914453,-0.0010608789606638,
0.00229621243031557));
#25241=CARTESIAN_POINT('Ctrl Pts',(-0.238020387591146,-0.00106084120527947,
0.00230090505063957));
#25242=CARTESIAN_POINT('Ctrl Pts',(-0.238020352159595,-0.00106079956502891,
0.00230559488122262));
#25243=CARTESIAN_POINT('Ctrl Pts',(-0.238020316619799,-0.00106075405521242,
0.0023102818979168));
#25244=CARTESIAN_POINT('',(-0.238020316532523,0.0160607545725048,-0.00231025307801074));
#25245=CARTESIAN_POINT('Ctrl Pts',(-0.238020318599054,0.0160609816928344,
-0.00231040371569625));
#25246=CARTESIAN_POINT('Ctrl Pts',(-0.238014604517819,0.016053500205237,
-0.00306190043396615));
#25247=CARTESIAN_POINT('Ctrl Pts',(-0.238004107699624,0.0158415514403933,
-0.00446246711947055));
#25248=CARTESIAN_POINT('Ctrl Pts',(-0.237993318103923,0.0152778506838575,
-0.00587614646494471));
#25249=CARTESIAN_POINT('Ctrl Pts',(-0.237986081901558,0.0147484689245685,
-0.00680176347060161));
#25250=CARTESIAN_POINT('Ctrl Pts',(-0.23798136150549,0.0143340090615772,
-0.00739703324374946));
#25251=CARTESIAN_POINT('Ctrl Pts',(-0.237977986253456,0.0139854138410196,
-0.00781963052493187));
#25252=CARTESIAN_POINT('Ctrl Pts',(-0.237975976938392,0.0137543357831049,
-0.0080725654215816));
#25253=CARTESIAN_POINT('Ctrl Pts',(-0.237974841983293,0.0136151820866611,
-0.00821658632941533));
#25254=CARTESIAN_POINT('Ctrl Pts',(-0.237974243379501,0.0135400220076929,
-0.00829300142009656));
#25255=CARTESIAN_POINT('Ctrl Pts',(-0.237972889875128,0.0133608675439882,
-0.00846684804851594));
#25256=CARTESIAN_POINT('Ctrl Pts',(-0.237971411861785,0.0131526205788322,
-0.0086569885059668));
#25257=CARTESIAN_POINT('Ctrl Pts',(-0.237968828324772,0.0127606952743352,
-0.00899010162830897));
#25258=CARTESIAN_POINT('Ctrl Pts',(-0.23796558142955,0.0121803403678554,
-0.00940998980172909));
#25259=CARTESIAN_POINT('Ctrl Pts',(-0.237962258740912,0.011442842468399,
-0.00983942706026314));
#25260=CARTESIAN_POINT('Ctrl Pts',(-0.237958641690952,0.0104233649905898,
-0.010304854326046));
#25261=CARTESIAN_POINT('Ctrl Pts',(-0.237955622814505,0.00909678549852576,
-0.0106872846852435));
#25262=CARTESIAN_POINT('Ctrl Pts',(-0.237954410173046,0.00750600282866814,
-0.0108341606636561));
#25263=CARTESIAN_POINT('Ctrl Pts',(-0.237955607770554,0.00591243383673865,
-0.0106891746012175));
#25264=CARTESIAN_POINT('Ctrl Pts',(-0.237958618664386,0.00458475323403587,
-0.0103078244918697));
#25265=CARTESIAN_POINT('Ctrl Pts',(-0.237962231319832,0.00356398336301219,
-0.00984298458230142));
#25266=CARTESIAN_POINT('Ctrl Pts',(-0.237965551695216,0.00282554706414488,
-0.00941384981571709));
#25267=CARTESIAN_POINT('Ctrl Pts',(-0.237968797940997,0.00224435283945219,
-0.00899403466574531));
#25268=CARTESIAN_POINT('Ctrl Pts',(-0.237971380735772,0.00185193966955052,
-0.00866100194975026));
#25269=CARTESIAN_POINT('Ctrl Pts',(-0.237972859646126,0.00164327921911097,
-0.00847073517420804));
#25270=CARTESIAN_POINT('Ctrl Pts',(-0.237974210547823,0.00146420766709804,
-0.00829721467232998));
#25271=CARTESIAN_POINT('Ctrl Pts',(-0.237974819394004,0.00138764039313657,
-0.00821947035633698));
#25272=CARTESIAN_POINT('Ctrl Pts',(-0.237975950670599,0.00124880288754097,
-0.0080759099575687));
#25273=CARTESIAN_POINT('Ctrl Pts',(-0.237977961897761,0.00101723345554436,
-0.00782271998155836));
#25274=CARTESIAN_POINT('Ctrl Pts',(-0.237981336299155,0.000668421674808697,
-0.00740024611366686));
#25275=CARTESIAN_POINT('Ctrl Pts',(-0.237986058550236,0.000253414863704401,
-0.00680477583222583));
#25276=CARTESIAN_POINT('Ctrl Pts',(-0.237993298003416,-0.000276649707725574,
-0.0058787917379549));
#25277=CARTESIAN_POINT('Ctrl Pts',(-0.238004094529999,-0.000841198091866792,
-0.00446423767063164));
#25278=CARTESIAN_POINT('Ctrl Pts',(-0.238014599650372,-0.00105349359705469,
-0.00306254026317131));
#25279=CARTESIAN_POINT('Ctrl Pts',(-0.23802031859663,-0.00106098145426406,
-0.00231040371318102));
#25280=CARTESIAN_POINT('Ctrl Pts',(-0.238020422914454,0.0160608789606638,
0.00229621243031557));
#25281=CARTESIAN_POINT('Ctrl Pts',(-0.238023371086056,0.0160640301194921,
0.00190455459861773));
#25282=CARTESIAN_POINT('Ctrl Pts',(-0.238025565230504,0.0160667702507188,
0.00151323660130437));
#25283=CARTESIAN_POINT('Ctrl Pts',(-0.238027005347798,0.0160686427431678,
0.00112190150667837));
#25284=CARTESIAN_POINT('Ctrl Pts',(-0.238028380588605,0.0160704308808675,
0.000748195841645495));
#25285=CARTESIAN_POINT('Ctrl Pts',(-0.238029068209008,0.0160714200523582,
0.000374041179736735));
#25286=CARTESIAN_POINT('Ctrl Pts',(-0.238029068209008,0.0160714200523582,
5.20127317150229E-18));
#25287=CARTESIAN_POINT('Ctrl Pts',(-0.238029068209007,0.0160714200523582,
-0.00037404117967552));
#25288=CARTESIAN_POINT('Ctrl Pts',(-0.238028380588604,0.0160704308808678,
-0.000748195841581645));
#25289=CARTESIAN_POINT('Ctrl Pts',(-0.238027005347796,0.0160686427431678,
-0.00112190150667836));
#25290=CARTESIAN_POINT('Ctrl Pts',(-0.238025565230502,0.0160667702507193,
-0.00151323660122079));
#25291=CARTESIAN_POINT('Ctrl Pts',(-0.238023371086054,0.0160640301194929,
-0.00190455459852223));
#25292=CARTESIAN_POINT('Ctrl Pts',(-0.238020422914453,0.0160608789606638,
-0.00229621243031559));
#25293=CARTESIAN_POINT('Ctrl Pts',(-0.238020387591146,0.0160608412052795,
-0.00230090505064033));
#25294=CARTESIAN_POINT('Ctrl Pts',(-0.238020352159595,0.0160607995650289,
-0.00230559488122414));
#25295=CARTESIAN_POINT('Ctrl Pts',(-0.238020316619799,0.0160607540552124,
-0.00231028189791906));
#25296=CARTESIAN_POINT('Origin',(-0.24,0.0075,0.));
#25297=CARTESIAN_POINT('',(-0.1795,0.0075,0.005));
#25298=CARTESIAN_POINT('',(-0.1795,0.0075,-0.005));
#25299=CARTESIAN_POINT('Origin',(-0.1795,0.0075,0.));
#25300=CARTESIAN_POINT('Origin',(-0.1795,0.0075,0.));
#25301=CARTESIAN_POINT('',(-0.1405,0.0075,0.005));
#25302=CARTESIAN_POINT('',(-0.24,0.0075,0.005));
#25303=CARTESIAN_POINT('',(-0.1405,0.0075,-0.005));
#25304=CARTESIAN_POINT('Origin',(-0.1405,0.0075,0.));
#25305=CARTESIAN_POINT('Origin',(-0.1405,0.0075,0.));
#25306=CARTESIAN_POINT('Origin',(-0.24,0.0075,0.));
#25307=CARTESIAN_POINT('',(-0.16,0.0075,0.0074756477610481));
#25308=CARTESIAN_POINT('Origin',(-0.16,0.0075,0.));
#25309=CARTESIAN_POINT('',(-0.1795,0.0075,0.0074756477610481));
#25310=CARTESIAN_POINT('',(-0.24,0.0075,0.0074756477610481));
#25311=CARTESIAN_POINT('',(-0.1795,0.0075,-0.0074756477610481));
#25312=CARTESIAN_POINT('Origin',(-0.1795,0.0075,0.));
#25313=CARTESIAN_POINT('Origin',(-0.1795,0.0075,0.));
#25314=CARTESIAN_POINT('Origin',(-0.16,0.0075,0.));
#25315=CARTESIAN_POINT('',(-0.1405,0.0075,0.00932888901198444));
#25316=CARTESIAN_POINT('',(-0.1405,0.0075,-0.00932888901198444));
#25317=CARTESIAN_POINT('Origin',(-0.1405,0.0075,0.));
#25318=CARTESIAN_POINT('Origin',(-0.1405,0.0075,0.));
#25319=CARTESIAN_POINT('',(-0.1406,0.0075,0.00932888901198444));
#25320=CARTESIAN_POINT('',(-0.16,0.0075,0.00932888901198444));
#25321=CARTESIAN_POINT('',(-0.1406,0.0075,-0.00932888901198444));
#25322=CARTESIAN_POINT('Origin',(-0.1406,0.0075,0.));
#25323=CARTESIAN_POINT('Origin',(-0.1406,0.0075,0.));
#25324=CARTESIAN_POINT('Origin',(-0.16,0.0075,0.));
#25325=CARTESIAN_POINT('',(-0.159473534924936,0.0075,0.00932888901198444));
#25326=CARTESIAN_POINT('Origin',(-0.159473534924936,0.0075,0.));
#25327=CARTESIAN_POINT('',(-0.1595,0.0075,0.00932888901198444));
#25328=CARTESIAN_POINT('',(-0.16,0.0075,0.00932888901198444));
#25329=CARTESIAN_POINT('',(-0.1595,0.0075,-0.00932888901198444));
#25330=CARTESIAN_POINT('Origin',(-0.1595,0.0075,0.));
#25331=CARTESIAN_POINT('Origin',(-0.1595,0.0075,0.));
#25332=CARTESIAN_POINT('Origin',(-0.14,0.,0.));
#25333=CARTESIAN_POINT('',(-0.14,0.0075,-0.00882888901198444));
#25334=CARTESIAN_POINT('Origin',(-0.14,0.0075,0.));
#25335=CARTESIAN_POINT('',(-0.14,0.0075,-0.0055));
#25336=CARTESIAN_POINT('Origin',(-0.14,0.0075,0.));
#25337=CARTESIAN_POINT('Origin',(-0.16,0.,0.));
#25338=CARTESIAN_POINT('',(-0.16,0.0075,-0.00882888901198444));
#25339=CARTESIAN_POINT('Origin',(-0.16,0.0075,0.));
#25340=CARTESIAN_POINT('Origin',(0.0540947251599426,0.0075,0.));
#25341=CARTESIAN_POINT('',(-0.1585,0.0075,-0.00898940279602035));
#25342=CARTESIAN_POINT('',(-0.1585,0.0075,0.00898940279602035));
#25343=CARTESIAN_POINT('Origin',(-0.1585,0.0075,0.));
#25344=CARTESIAN_POINT('Origin',(-0.1585,0.0075,0.));
#25345=CARTESIAN_POINT('',(-0.159,0.0075,0.00898940279602035));
#25346=CARTESIAN_POINT('',(0.0540947251599426,0.0075,0.00898940279602035));
#25347=CARTESIAN_POINT('Origin',(-0.159,0.0075,0.));
#25348=CARTESIAN_POINT('Origin',(0.0540947251599426,0.0075,0.));
#25349=CARTESIAN_POINT('',(-0.141,0.0075,-0.00912888901198444));
#25350=CARTESIAN_POINT('',(-0.141,0.0075,0.00912888901198444));
#25351=CARTESIAN_POINT('Origin',(-0.141,0.0075,0.));
#25352=CARTESIAN_POINT('Origin',(-0.141,0.0075,0.));
#25353=CARTESIAN_POINT('',(-0.1415,0.0075,0.00912888901198444));
#25354=CARTESIAN_POINT('',(0.0540947251599426,0.0075,0.00912888901198444));
#25355=CARTESIAN_POINT('Origin',(-0.1415,0.0075,0.));
#25356=CARTESIAN_POINT('Origin',(-0.16,0.0075,0.));
#25357=CARTESIAN_POINT('',(-0.150973534924937,0.0075,0.00932888901198444));
#25358=CARTESIAN_POINT('Origin',(-0.150973534924937,0.0075,0.));
#25359=CARTESIAN_POINT('',(-0.158026465075064,0.0075,0.00932888901198444));
#25360=CARTESIAN_POINT('',(-0.16,0.0075,0.00932888901198444));
#25361=CARTESIAN_POINT('',(-0.158026465075064,0.0075,-0.00932888901198444));
#25362=CARTESIAN_POINT('Origin',(-0.158026465075064,0.0075,0.));
#25363=CARTESIAN_POINT('Origin',(-0.158026465075064,0.0075,0.));
#25364=CARTESIAN_POINT('Origin',(-0.16,0.0075,0.));
#25365=CARTESIAN_POINT('',(-0.1419,0.0075,0.00932888901198444));
#25366=CARTESIAN_POINT('Origin',(-0.1419,0.0075,0.));
#25367=CARTESIAN_POINT('',(-0.1421,0.0075,0.00932888901198444));
#25368=CARTESIAN_POINT('',(-0.16,0.0075,0.00932888901198444));
#25369=CARTESIAN_POINT('',(-0.1421,0.0075,-0.00932888901198444));
#25370=CARTESIAN_POINT('Origin',(-0.1421,0.0075,0.));
#25371=CARTESIAN_POINT('Origin',(-0.1421,0.0075,0.));
#25372=CARTESIAN_POINT('Origin',(0.0540947251599426,0.0075,0.));
#25373=CARTESIAN_POINT('',(-0.15,0.0075,-0.00898940279602035));
#25374=CARTESIAN_POINT('',(-0.15,0.0075,0.00898940279602035));
#25375=CARTESIAN_POINT('Origin',(-0.15,0.0075,0.));
#25376=CARTESIAN_POINT('Origin',(-0.15,0.0075,0.));
#25377=CARTESIAN_POINT('',(-0.1505,0.0075,0.00898940279602035));
#25378=CARTESIAN_POINT('',(0.0540947251599426,0.0075,0.00898940279602035));
#25379=CARTESIAN_POINT('Origin',(-0.1505,0.0075,0.));
#25380=CARTESIAN_POINT('Origin',(0.0540947251599426,0.0075,0.));
#25381=CARTESIAN_POINT('',(-0.1425,0.0075,-0.00912888901198443));
#25382=CARTESIAN_POINT('',(-0.1425,0.0075,0.00912888901198443));
#25383=CARTESIAN_POINT('Origin',(-0.1425,0.0075,0.));
#25384=CARTESIAN_POINT('Origin',(-0.1425,0.0075,0.));
#25385=CARTESIAN_POINT('',(-0.143,0.0075,0.00912888901198443));
#25386=CARTESIAN_POINT('',(0.0540947251599426,0.0075,0.00912888901198443));
#25387=CARTESIAN_POINT('Origin',(-0.143,0.0075,0.));
#25388=CARTESIAN_POINT('Origin',(-0.16,0.0075,0.));
#25389=CARTESIAN_POINT('',(-0.1479,0.0075,0.00932888901198444));
#25390=CARTESIAN_POINT('Origin',(-0.1479,0.0075,0.));
#25391=CARTESIAN_POINT('',(-0.149526465075064,0.0075,0.00932888901198444));
#25392=CARTESIAN_POINT('',(-0.16,0.0075,0.00932888901198444));
#25393=CARTESIAN_POINT('',(-0.149526465075064,0.0075,-0.00932888901198444));
#25394=CARTESIAN_POINT('Origin',(-0.149526465075064,0.0075,0.));
#25395=CARTESIAN_POINT('Origin',(-0.149526465075064,0.0075,0.));
#25396=CARTESIAN_POINT('Origin',(0.0540947251599426,0.0075,0.));
#25397=CARTESIAN_POINT('',(-0.147,0.0075,-0.0091288890119844));
#25398=CARTESIAN_POINT('',(-0.147,0.0075,0.0091288890119844));
#25399=CARTESIAN_POINT('Origin',(-0.147,0.0075,0.));
#25400=CARTESIAN_POINT('Origin',(-0.147,0.0075,0.));
#25401=CARTESIAN_POINT('',(-0.1475,0.0075,0.0091288890119844));
#25402=CARTESIAN_POINT('',(0.0540947251599426,0.0075,0.0091288890119844));
#25403=CARTESIAN_POINT('Origin',(-0.1475,0.0075,0.));
#25404=CARTESIAN_POINT('Origin',(-0.16,0.0075,0.));
#25405=CARTESIAN_POINT('',(-0.1464,0.0075,0.00932888901198444));
#25406=CARTESIAN_POINT('Origin',(-0.1464,0.0075,0.));
#25407=CARTESIAN_POINT('',(-0.1466,0.0075,0.00932888901198444));
#25408=CARTESIAN_POINT('',(-0.16,0.0075,0.00932888901198444));
#25409=CARTESIAN_POINT('',(-0.1466,0.0075,-0.00932888901198444));
#25410=CARTESIAN_POINT('Origin',(-0.1466,0.0075,0.));
#25411=CARTESIAN_POINT('Origin',(-0.1466,0.0075,0.));
#25412=CARTESIAN_POINT('Origin',(0.0540947251599426,0.0075,0.));
#25413=CARTESIAN_POINT('',(-0.1455,0.0075,-0.00912888901198441));
#25414=CARTESIAN_POINT('',(-0.1455,0.0075,0.00912888901198441));
#25415=CARTESIAN_POINT('Origin',(-0.1455,0.0075,0.));
#25416=CARTESIAN_POINT('Origin',(-0.1455,0.0075,0.));
#25417=CARTESIAN_POINT('',(-0.146,0.0075,0.00912888901198441));
#25418=CARTESIAN_POINT('',(0.0540947251599426,0.0075,0.00912888901198441));
#25419=CARTESIAN_POINT('Origin',(-0.146,0.0075,0.));
#25420=CARTESIAN_POINT('Origin',(-0.16,0.0075,0.));
#25421=CARTESIAN_POINT('',(-0.1449,0.0075,0.00932888901198444));
#25422=CARTESIAN_POINT('Origin',(-0.1449,0.0075,0.));
#25423=CARTESIAN_POINT('',(-0.1451,0.0075,0.00932888901198444));
#25424=CARTESIAN_POINT('',(-0.16,0.0075,0.00932888901198444));
#25425=CARTESIAN_POINT('',(-0.1451,0.0075,-0.00932888901198444));
#25426=CARTESIAN_POINT('Origin',(-0.1451,0.0075,0.));
#25427=CARTESIAN_POINT('Origin',(-0.1451,0.0075,0.));
#25428=CARTESIAN_POINT('Origin',(0.0540947251599426,0.0075,0.));
#25429=CARTESIAN_POINT('',(-0.144,0.0075,-0.00912888901198442));
#25430=CARTESIAN_POINT('',(-0.144,0.0075,0.00912888901198442));
#25431=CARTESIAN_POINT('Origin',(-0.144,0.0075,0.));
#25432=CARTESIAN_POINT('Origin',(-0.144,0.0075,0.));
#25433=CARTESIAN_POINT('',(-0.1445,0.0075,0.00912888901198442));
#25434=CARTESIAN_POINT('',(0.0540947251599426,0.0075,0.00912888901198442));
#25435=CARTESIAN_POINT('Origin',(-0.1445,0.0075,0.));
#25436=CARTESIAN_POINT('Origin',(-0.16,0.0075,0.));
#25437=CARTESIAN_POINT('',(-0.1434,0.0075,0.00932888901198444));
#25438=CARTESIAN_POINT('Origin',(-0.1434,0.0075,0.));
#25439=CARTESIAN_POINT('',(-0.1436,0.0075,0.00932888901198444));
#25440=CARTESIAN_POINT('',(-0.16,0.0075,0.00932888901198444));
#25441=CARTESIAN_POINT('',(-0.1436,0.0075,-0.00932888901198444));
#25442=CARTESIAN_POINT('Origin',(-0.1436,0.0075,0.));
#25443=CARTESIAN_POINT('Origin',(-0.1436,0.0075,0.));
#25444=CARTESIAN_POINT('Ctrl Pts',(-0.238376419148325,0.0160572510994551,
0.00229523935965256));
#25445=CARTESIAN_POINT('Ctrl Pts',(-0.180143329927774,0.0166506887410553,
0.00245441214111993));
#25446=CARTESIAN_POINT('Ctrl Pts',(-0.238376419148325,0.0160499153270237,
0.00339695540894448));
#25447=CARTESIAN_POINT('Ctrl Pts',(-0.180143329927774,0.0163802403000704,
0.00346535234146251));
#25448=CARTESIAN_POINT('Ctrl Pts',(-0.238376419148325,0.0156043581343594,
0.00560766010208411));
#25449=CARTESIAN_POINT('Ctrl Pts',(-0.180143329927774,0.0155045639563625,
0.00538672371465897));
#25450=CARTESIAN_POINT('Ctrl Pts',(-0.238376419148325,0.0137116283891667,
0.00844195664423076));
#25451=CARTESIAN_POINT('Ctrl Pts',(-0.180143329927774,0.0133464539612027,
0.00767441593321455));
#25452=CARTESIAN_POINT('Ctrl Pts',(-0.238376419148325,0.0108665999736013,
0.0103474435450232));
#25453=CARTESIAN_POINT('Ctrl Pts',(-0.180143329927774,0.0105817751956803,
0.00914209790934899));
#25454=CARTESIAN_POINT('Ctrl Pts',(-0.238376419148325,0.0075,0.0110189940848823));
#25455=CARTESIAN_POINT('Ctrl Pts',(-0.180143329927774,0.0075,0.00964748427001006));
#25456=CARTESIAN_POINT('Ctrl Pts',(-0.238376419148325,0.00413340002639867,
0.0103474435450232));
#25457=CARTESIAN_POINT('Ctrl Pts',(-0.180143329927774,0.0044182248043197,
0.00914209790934899));
#25458=CARTESIAN_POINT('Ctrl Pts',(-0.238376419148325,0.00128837161083331,
0.00844195664423074));
#25459=CARTESIAN_POINT('Ctrl Pts',(-0.180143329927774,0.00165354603879735,
0.00767441593321453));
#25460=CARTESIAN_POINT('Ctrl Pts',(-0.238376419148325,-0.000604358134359394,
0.00560766010208411));
#25461=CARTESIAN_POINT('Ctrl Pts',(-0.180143329927774,-0.000504563956362522,
0.00538672371465897));
#25462=CARTESIAN_POINT('Ctrl Pts',(-0.238376419148325,-0.00104991532702373,
0.00339695540894447));
#25463=CARTESIAN_POINT('Ctrl Pts',(-0.180143329927774,-0.00138024030007043,
0.00346535234146251));
#25464=CARTESIAN_POINT('Ctrl Pts',(-0.238376419148325,-0.00105996989569538,
0.00188691951593846));
#25465=CARTESIAN_POINT('Ctrl Pts',(-0.180143329927774,-0.00175092279430951,
0.00207973579427586));
#25466=CARTESIAN_POINT('Ctrl Pts',(-0.238376419148325,-0.00106440179407383,
0.00111305841215638));
#25467=CARTESIAN_POINT('Ctrl Pts',(-0.180143329927774,-0.00191431390523475,
0.0012839986244053));
#25468=CARTESIAN_POINT('Ctrl Pts',(-0.238376419148325,-0.00106680965804379,
-1.88715094039015E-18));
#25469=CARTESIAN_POINT('Ctrl Pts',(-0.180143329927774,-0.00200308479649061,
-3.46556198647675E-18));
#25470=CARTESIAN_POINT('Ctrl Pts',(-0.238376419148325,-0.00106440179407383,
-0.00111305841215639));
#25471=CARTESIAN_POINT('Ctrl Pts',(-0.180143329927774,-0.00191431390523475,
-0.0012839986244053));
#25472=CARTESIAN_POINT('Ctrl Pts',(-0.238376419148325,-0.00105996989569538,
-0.00188691951593846));
#25473=CARTESIAN_POINT('Ctrl Pts',(-0.180143329927774,-0.00175092279430951,
-0.00207973579427587));
#25474=CARTESIAN_POINT('Ctrl Pts',(-0.238376419148325,-0.00104991532702373,
-0.00339695540894448));
#25475=CARTESIAN_POINT('Ctrl Pts',(-0.180143329927774,-0.00138024030007042,
-0.00346535234146251));
#25476=CARTESIAN_POINT('Ctrl Pts',(-0.238376419148325,-0.000604358134359395,
-0.00560766010208411));
#25477=CARTESIAN_POINT('Ctrl Pts',(-0.180143329927774,-0.000504563956362519,
-0.00538672371465899));
#25478=CARTESIAN_POINT('Ctrl Pts',(-0.238376419148325,0.00128837161083331,
-0.00844195664423075));
#25479=CARTESIAN_POINT('Ctrl Pts',(-0.180143329927774,0.00165354603879737,
-0.00767441593321454));
#25480=CARTESIAN_POINT('Ctrl Pts',(-0.238376419148325,0.00413340002639866,
-0.0103474435450231));
#25481=CARTESIAN_POINT('Ctrl Pts',(-0.180143329927774,0.0044182248043197,
-0.00914209790934901));
#25482=CARTESIAN_POINT('Ctrl Pts',(-0.238376419148325,0.0075,-0.0110189940848823));
#25483=CARTESIAN_POINT('Ctrl Pts',(-0.180143329927774,0.0075,-0.00964748427001004));
#25484=CARTESIAN_POINT('Ctrl Pts',(-0.238376419148325,0.0108665999736013,
-0.0103474435450232));
#25485=CARTESIAN_POINT('Ctrl Pts',(-0.180143329927774,0.0105817751956803,
-0.00914209790934901));
#25486=CARTESIAN_POINT('Ctrl Pts',(-0.238376419148325,0.0137116283891667,
-0.00844195664423074));
#25487=CARTESIAN_POINT('Ctrl Pts',(-0.180143329927774,0.0133464539612027,
-0.00767441593321454));
#25488=CARTESIAN_POINT('Ctrl Pts',(-0.238376419148325,0.0156043581343594,
-0.00560766010208412));
#25489=CARTESIAN_POINT('Ctrl Pts',(-0.180143329927774,0.0155045639563625,
-0.00538672371465897));
#25490=CARTESIAN_POINT('Ctrl Pts',(-0.238376419148325,0.0160499153270237,
-0.00339695540894448));
#25491=CARTESIAN_POINT('Ctrl Pts',(-0.180143329927774,0.0163802403000704,
-0.00346535234146251));
#25492=CARTESIAN_POINT('Ctrl Pts',(-0.238376419148325,0.0160599698956954,
-0.00188691951593846));
#25493=CARTESIAN_POINT('Ctrl Pts',(-0.180143329927774,0.0167509227943095,
-0.00207973579427587));
#25494=CARTESIAN_POINT('Ctrl Pts',(-0.238376419148325,0.0160644017940738,
-0.00111305841215638));
#25495=CARTESIAN_POINT('Ctrl Pts',(-0.180143329927774,0.0169143139052348,
-0.0012839986244053));
#25496=CARTESIAN_POINT('Ctrl Pts',(-0.238376419148325,0.0160668096580438,
-5.5742513075403E-20));
#25497=CARTESIAN_POINT('Ctrl Pts',(-0.180143329927774,0.0170030847964906,
-2.05506317145176E-18));
#25498=CARTESIAN_POINT('Ctrl Pts',(-0.238376419148325,0.0160644017940738,
0.00111305841215638));
#25499=CARTESIAN_POINT('Ctrl Pts',(-0.180143329927774,0.0169143139052348,
0.0012839986244053));
#25500=CARTESIAN_POINT('Ctrl Pts',(-0.238376419148325,0.0160599698956954,
0.00188691951593846));
#25501=CARTESIAN_POINT('Ctrl Pts',(-0.180143329927774,0.0167509227943095,
0.00207973579427586));
#25502=CARTESIAN_POINT('Ctrl Pts',(-0.238376419148325,0.0160572510994551,
0.00229523935965256));
#25503=CARTESIAN_POINT('Ctrl Pts',(-0.180143329927774,0.0166506887410553,
0.00245441214111993));
#25504=CARTESIAN_POINT('',(-0.238020316532543,0.0160607545725302,0.00231025307448946));
#25505=CARTESIAN_POINT('Ctrl Pts',(-0.238020316619822,0.0160607540552411,
0.00231028189496567));
#25506=CARTESIAN_POINT('Ctrl Pts',(-0.23802035215961,0.0160607995650464,
0.00230559487925404));
#25507=CARTESIAN_POINT('Ctrl Pts',(-0.238020387591155,0.0160608412052874,
0.0023009050496547));
#25508=CARTESIAN_POINT('Ctrl Pts',(-0.238020422914454,0.0160608789606638,
0.00229621243031557));
#25509=CARTESIAN_POINT('Ctrl Pts',(-0.237977937649492,0.00102548423602743,
0.00782605181637851));
#25510=CARTESIAN_POINT('Ctrl Pts',(-0.237977771361891,0.00104352664243288,
0.0078469252176614));
#25511=CARTESIAN_POINT('Ctrl Pts',(-0.237976990708435,0.00112907719101165,
0.00794495085130883));
#25512=CARTESIAN_POINT('Ctrl Pts',(-0.237975976937705,0.0012456642779511,
0.00807256548637949));
#25513=CARTESIAN_POINT('Ctrl Pts',(-0.237974841982942,0.00138481794771289,
0.00821658636396061));
#25514=CARTESIAN_POINT('Ctrl Pts',(-0.237974243379628,0.00145997797384131,
0.00829300140192245));
#25515=CARTESIAN_POINT('Ctrl Pts',(-0.237972889874965,0.00163913249662495,
0.00846684808778011));
#25516=CARTESIAN_POINT('Ctrl Pts',(-0.237971411861517,0.00184737950156088,
0.00865698857652469));
#25517=CARTESIAN_POINT('Ctrl Pts',(-0.237968828324226,0.00223930487946204,
0.00899010176098222));
#25518=CARTESIAN_POINT('Ctrl Pts',(-0.237965581428728,0.00281965996064833,
0.0094099899606304));
#25519=CARTESIAN_POINT('Ctrl Pts',(-0.237962258739981,0.00355715761932815,
0.00983942728785487));
#25520=CARTESIAN_POINT('Ctrl Pts',(-0.237958641689478,0.00457663675962997,
0.0103048542155954));
#25521=CARTESIAN_POINT('Ctrl Pts',(-0.237955622816736,0.00590320392835369,
0.0106872867840954));
#25522=CARTESIAN_POINT('Ctrl Pts',(-0.237954410161632,0.00749403703264914,
0.0108341531591348));
#25523=CARTESIAN_POINT('Ctrl Pts',(-0.23795560781398,0.00908741729428714,
0.0106892025204542));
#25524=CARTESIAN_POINT('Ctrl Pts',(-0.237958618842412,0.0104152747494254,
0.0103078197503335));
#25525=CARTESIAN_POINT('Ctrl Pts',(-0.237962231600465,0.0114360766911925,
0.00984295543332729));
#25526=CARTESIAN_POINT('Ctrl Pts',(-0.237965552197248,0.0121745503730158,
0.00941378412783473));
#25527=CARTESIAN_POINT('Ctrl Pts',(-0.237968798249626,0.0127557129303162,
0.00899399101451944));
#25528=CARTESIAN_POINT('Ctrl Pts',(-0.2379713816927,0.0131481981613132,
0.00866087544582393));
#25529=CARTESIAN_POINT('Ctrl Pts',(-0.237972859766266,0.0133567445403098,
0.00847071847746978));
#25530=CARTESIAN_POINT('Ctrl Pts',(-0.237974213449617,0.0135361635963531,
0.00829684006850807));
#25531=CARTESIAN_POINT('Ctrl Pts',(-0.237974812051711,0.0136114201539808,
0.00822042272077482));
#25532=CARTESIAN_POINT('Ctrl Pts',(-0.237975947163907,0.0137507676709391,
0.00807638082371326));
#25533=CARTESIAN_POINT('Ctrl Pts',(-0.237977956915679,0.0139821694340823,
0.00782339731578715));
#25534=CARTESIAN_POINT('Ctrl Pts',(-0.237981333384561,0.014331271685258,
0.00740067143450062));
#25535=CARTESIAN_POINT('Ctrl Pts',(-0.2379860561487,0.0147463578891999,
0.00680513776468162));
#25536=CARTESIAN_POINT('Ctrl Pts',(-0.237993296733614,0.0152765669110609,
0.00587899756444639));
#25537=CARTESIAN_POINT('Ctrl Pts',(-0.238004094098004,0.0158411892598538,
0.00446430697140144));
#25538=CARTESIAN_POINT('Ctrl Pts',(-0.238014599575372,0.0160534934989504,
0.00306255012693011));
#25539=CARTESIAN_POINT('Ctrl Pts',(-0.238020318596638,0.0160609814542743,
0.00231040371210835));
#25540=CARTESIAN_POINT('Ctrl Pts',(-0.180494077221453,0.00130607217168702,
0.00717829214732417));
#25541=CARTESIAN_POINT('Ctrl Pts',(-0.180493592787613,0.0015545815750099,
0.00739357222966939));
#25542=CARTESIAN_POINT('Ctrl Pts',(-0.180493140404119,0.00181416743482917,
0.00759583454647146));
#25543=CARTESIAN_POINT('Ctrl Pts',(-0.180492713748997,0.00208357848608163,
0.00778381456156277));
#25544=CARTESIAN_POINT('Origin',(-0.18,0.0075,0.));
#25545=CARTESIAN_POINT('',(-0.18000000007387,0.00163316081088028,0.00680057000546517));
#25546=CARTESIAN_POINT('Ctrl Pts',(-0.18000000007387,0.00163316081088028,
0.00680057000546517));
#25547=CARTESIAN_POINT('Ctrl Pts',(-0.180000000073869,0.00163311910190787,
0.0068005338709428));
#25548=CARTESIAN_POINT('Ctrl Pts',(-0.180000000073867,0.00163307739326464,
0.00680049773603036));
#25549=CARTESIAN_POINT('Ctrl Pts',(-0.180000000073866,0.00163303568495152,
0.0068004616007287));
#25550=CARTESIAN_POINT('Ctrl Pts',(-0.180000000092441,0.002369415201346,
0.00737400928367846));
#25551=CARTESIAN_POINT('Ctrl Pts',(-0.180000000083634,0.00211429283077817,
0.0071959755706896));
#25552=CARTESIAN_POINT('Ctrl Pts',(-0.180000000081285,0.00186847253526104,
0.00700443205911563));
#25553=CARTESIAN_POINT('Ctrl Pts',(-0.18000000007387,0.00163316081088028,
0.00680057000546517));
#25554=CARTESIAN_POINT('',(-0.18,0.0075,-0.0079756477610481));
#25555=CARTESIAN_POINT('Origin',(-0.18,0.0075,0.));
#25556=CARTESIAN_POINT('Origin',(-0.18,0.0075,0.));
#25557=CARTESIAN_POINT('',(-0.18,0.0075,-0.0045));
#25558=CARTESIAN_POINT('Origin',(-0.18,0.0075,0.));
#25559=CARTESIAN_POINT('Origin',(-0.24,0.,0.));
#25560=CARTESIAN_POINT('',(-0.239999990168078,0.00093904782781612,0.00229080150890899));
#25561=CARTESIAN_POINT('',(-0.239999990171285,0.014060952172193,0.00229080150799885));
#25562=CARTESIAN_POINT('Ctrl Pts',(-0.239999996094951,0.00093904787461105,
0.00229080150892728));
#25563=CARTESIAN_POINT('Ctrl Pts',(-0.239999997101475,0.000948692154517853,
0.00327481805300442));
#25564=CARTESIAN_POINT('Ctrl Pts',(-0.239999998053108,0.00118441104025385,
0.00425953843427544));
#25565=CARTESIAN_POINT('Ctrl Pts',(-0.239999998922749,0.00162324794014383,
0.00514324753713933));
#25566=CARTESIAN_POINT('Ctrl Pts',(-0.239999999559175,0.0019444000203298,
0.0057899684868479));
#25567=CARTESIAN_POINT('Ctrl Pts',(-0.240000000150506,0.00237305339304198,
0.00638245831932459));
#25568=CARTESIAN_POINT('Ctrl Pts',(-0.240000000595735,0.00288415377574258,
0.00688859824331171));
#25569=CARTESIAN_POINT('Ctrl Pts',(-0.240000001209158,0.00358833160940053,
0.0075859417148971));
#25570=CARTESIAN_POINT('Ctrl Pts',(-0.240000001652703,0.00445542634564925,
0.00812227657472353));
#25571=CARTESIAN_POINT('Ctrl Pts',(-0.240000002018159,0.00539660868660465,
0.00844062167001609));
#25572=CARTESIAN_POINT('Ctrl Pts',(-0.240000002280407,0.00607199510526324,
0.0086690640710804));
#25573=CARTESIAN_POINT('Ctrl Pts',(-0.240000002506559,0.00678456933559004,
0.00878605448646416));
#25574=CARTESIAN_POINT('Ctrl Pts',(-0.240000002526878,0.0074955997506256,
0.00878612424472651));
#25575=CARTESIAN_POINT('Ctrl Pts',(-0.240000002554858,0.00847475043474964,
0.00878622030791714));
#25576=CARTESIAN_POINT('Ctrl Pts',(-0.240000002171471,0.0094577774348298,
0.00856303209124745));
#25577=CARTESIAN_POINT('Ctrl Pts',(-0.24000000179428,0.0103436536206028,
0.00813712929230807));
#25578=CARTESIAN_POINT('Ctrl Pts',(-0.240000001515866,0.0109975392046676,
0.00782276064247662));
#25579=CARTESIAN_POINT('Ctrl Pts',(-0.240000001257246,0.0115982954087712,
0.00739923147750592));
#25580=CARTESIAN_POINT('Ctrl Pts',(-0.240000000602187,0.0121128505559814,
0.00689155983415775));
#25581=CARTESIAN_POINT('Ctrl Pts',(-0.239999999683774,0.0128342721152729,
0.00617978915119394));
#25582=CARTESIAN_POINT('Ctrl Pts',(-0.23999999880627,0.0133885130222018,
0.00529542721886552));
#25583=CARTESIAN_POINT('Ctrl Pts',(-0.23999999800924,0.0137149174458767,
0.00433101787474712));
#25584=CARTESIAN_POINT('Ctrl Pts',(-0.239999997467613,0.0139367276453739,
0.00367564737882222));
#25585=CARTESIAN_POINT('Ctrl Pts',(-0.239999996808942,0.0140541566258168,
0.00298415385504518));
#25586=CARTESIAN_POINT('Ctrl Pts',(-0.239999996099761,0.0140609521253968,
0.00229080150801713));
#25587=CARTESIAN_POINT('',(-0.23999999609495,0.0140609521253889,-0.00229080150892896));
#25588=CARTESIAN_POINT('Ctrl Pts',(-0.239999978314326,0.0140609521966072,
0.00229080150800877));
#25589=CARTESIAN_POINT('Ctrl Pts',(-0.239999982890083,0.0140623369804884,
0.00214950739022427));
#25590=CARTESIAN_POINT('Ctrl Pts',(-0.239999985886701,0.0140636860354097,
0.00198109906617924));
#25591=CARTESIAN_POINT('Ctrl Pts',(-0.23999998754503,0.0140649627233419,
0.00179251014277393));
#25592=CARTESIAN_POINT('Ctrl Pts',(-0.239999988374194,0.014065601067308,
0.00169821568107128));
#25593=CARTESIAN_POINT('Ctrl Pts',(-0.23999998888584,0.0140662213195413,
0.00159887606952855));
#25594=CARTESIAN_POINT('Ctrl Pts',(-0.239999989109537,0.0140668601072055,
0.00148755770124551));
#25595=CARTESIAN_POINT('Ctrl Pts',(-0.239999989333234,0.0140674988948697,
0.00137623933296246));
#25596=CARTESIAN_POINT('Ctrl Pts',(-0.23999998921348,0.0140681562179323,
0.0012529422079391));
#25597=CARTESIAN_POINT('Ctrl Pts',(-0.239999988915679,0.014068685563465,
0.00114540075377642));
#25598=CARTESIAN_POINT('Ctrl Pts',(-0.239999988617878,0.0140692149089978,
0.00103785929961375));
#25599=CARTESIAN_POINT('Ctrl Pts',(-0.239999988207469,0.0140696162771043,
0.000946073516311766));
#25600=CARTESIAN_POINT('Ctrl Pts',(-0.239999987775988,0.0140699738331671,
0.000851201366531044));
#25601=CARTESIAN_POINT('Ctrl Pts',(-0.239999987344506,0.0140703313892298,
0.000756329216750322));
#25602=CARTESIAN_POINT('Ctrl Pts',(-0.239999986868716,0.0140706451332085,
0.00065837070049086));
#25603=CARTESIAN_POINT('Ctrl Pts',(-0.239999986453847,0.0140708940240656,
0.000562234778410537));
#25604=CARTESIAN_POINT('Ctrl Pts',(-0.239999985624108,0.0140713918057796,
0.00036996293424989));
#25605=CARTESIAN_POINT('Ctrl Pts',(-0.23999998509129,0.0140716301752879,
0.000184981466805796));
#25606=CARTESIAN_POINT('Ctrl Pts',(-0.23999998509129,0.014071630175288,
-4.55864146615709E-13));
#25607=CARTESIAN_POINT('Ctrl Pts',(-0.23999998509129,0.0140716301752881,
-0.000184981467717525));
#25608=CARTESIAN_POINT('Ctrl Pts',(-0.239999985624108,0.01407139180578,
-0.000369962934796753));
#25609=CARTESIAN_POINT('Ctrl Pts',(-0.239999986453847,0.0140708940240645,
-0.000562234779073522));
#25610=CARTESIAN_POINT('Ctrl Pts',(-0.239999986868716,0.0140706451332067,
-0.000658370701211906));
#25611=CARTESIAN_POINT('Ctrl Pts',(-0.239999987344507,0.0140703313892268,
-0.000756329217649677));
#25612=CARTESIAN_POINT('Ctrl Pts',(-0.239999987775988,0.0140699738331646,
-0.000851201367256255));
#25613=CARTESIAN_POINT('Ctrl Pts',(-0.23999998820747,0.0140696162771023,
-0.000946073516862834));
#25614=CARTESIAN_POINT('Ctrl Pts',(-0.239999988617878,0.014069214908998,
-0.00103785929963822));
#25615=CARTESIAN_POINT('Ctrl Pts',(-0.239999988915679,0.0140686855634605,
-0.00114540075468826));
#25616=CARTESIAN_POINT('Ctrl Pts',(-0.23999998921348,0.0140681562179229,
-0.00125294220973829));
#25617=CARTESIAN_POINT('Ctrl Pts',(-0.239999989333234,0.0140674988948486,
-0.00137623933706298));
#25618=CARTESIAN_POINT('Ctrl Pts',(-0.239999989109537,0.0140668601071775,
-0.00148755770664535));
#25619=CARTESIAN_POINT('Ctrl Pts',(-0.23999998888584,0.0140662213195064,
-0.00159887607622772));
#25620=CARTESIAN_POINT('Ctrl Pts',(-0.239999988374195,0.0140656010672713,
-0.00169821568806778));
#25621=CARTESIAN_POINT('Ctrl Pts',(-0.23999998754503,0.0140649627233053,
-0.00179251014966976));
#25622=CARTESIAN_POINT('Ctrl Pts',(-0.239999985886701,0.0140636860353734,
-0.00198109907287374));
#25623=CARTESIAN_POINT('Ctrl Pts',(-0.239999982890084,0.0140623369804603,
-0.00214950739512543));
#25624=CARTESIAN_POINT('Ctrl Pts',(-0.239999978314326,0.0140609521965983,
-0.00229080150892059));
#25625=CARTESIAN_POINT('',(-0.239999990171284,0.000939047827815039,-0.0022908015088178));
#25626=CARTESIAN_POINT('Ctrl Pts',(-0.23999999609495,0.0140609521253889,
-0.00229080150892896));
#25627=CARTESIAN_POINT('Ctrl Pts',(-0.239999997101474,0.0140513078454819,
-0.00327481805300426));
#25628=CARTESIAN_POINT('Ctrl Pts',(-0.239999998053107,0.0138155889597465,
-0.00425953843427357));
#25629=CARTESIAN_POINT('Ctrl Pts',(-0.239999998922749,0.0133767520598578,
-0.00514324753713624));
#25630=CARTESIAN_POINT('Ctrl Pts',(-0.239999999559175,0.0130555999797016,
-0.00578996848678572));
#25631=CARTESIAN_POINT('Ctrl Pts',(-0.240000000150506,0.0126269466070391,
-0.00638245831921348));
#25632=CARTESIAN_POINT('Ctrl Pts',(-0.240000000595735,0.0121158462244005,
-0.00688859824317014));
#25633=CARTESIAN_POINT('Ctrl Pts',(-0.240000001209157,0.0114116683907632,
-0.00758594171477775));
#25634=CARTESIAN_POINT('Ctrl Pts',(-0.240000001652703,0.0105445736545301,
-0.00812227657463066));
#25635=CARTESIAN_POINT('Ctrl Pts',(-0.240000002018158,0.0096033913135841,
-0.00844062166995183));
#25636=CARTESIAN_POINT('Ctrl Pts',(-0.240000002280407,0.00892800489499707,
-0.00866906407101473));
#25637=CARTESIAN_POINT('Ctrl Pts',(-0.240000002506559,0.00821543066474581,
-0.00878605448641982));
#25638=CARTESIAN_POINT('Ctrl Pts',(-0.240000002526877,0.00750440024977829,
-0.00878612424472624));
#25639=CARTESIAN_POINT('Ctrl Pts',(-0.240000002554857,0.0065252495656463,
-0.00878622030797757));
#25640=CARTESIAN_POINT('Ctrl Pts',(-0.240000002171471,0.00554222256554557,
-0.00856303209136526));
#25641=CARTESIAN_POINT('Ctrl Pts',(-0.240000001794279,0.00465634637974179,
-0.00813712929247474));
#25642=CARTESIAN_POINT('Ctrl Pts',(-0.240000001515865,0.00400246079572807,
-0.00782276064271482));
#25643=CARTESIAN_POINT('Ctrl Pts',(-0.240000001257246,0.0034017045916579,
-0.00739923147783583));
#25644=CARTESIAN_POINT('Ctrl Pts',(-0.240000000602186,0.00288714944445491,
-0.00689155983458874));
#25645=CARTESIAN_POINT('Ctrl Pts',(-0.239999999683773,0.00216572788509985,
-0.00617978915169404));
#25646=CARTESIAN_POINT('Ctrl Pts',(-0.239999998806269,0.00161148697809014,
-0.00529542721942));
#25647=CARTESIAN_POINT('Ctrl Pts',(-0.239999998009239,0.00128508255432472,
-0.00433101787533549));
#25648=CARTESIAN_POINT('Ctrl Pts',(-0.239999997467612,0.00106327235478633,
-0.00367564737949376));
#25649=CARTESIAN_POINT('Ctrl Pts',(-0.239999996808941,0.000945843374278495,
-0.00298415385579714));
#25650=CARTESIAN_POINT('Ctrl Pts',(-0.23999999609976,0.00093904787461117,
-0.00229080150883608));
#25651=CARTESIAN_POINT('Ctrl Pts',(-0.239999978314326,0.000939047803400774,
-0.00229080150882772));
#25652=CARTESIAN_POINT('Ctrl Pts',(-0.239999982890083,0.000937663019536478,
-0.00214950739458796));
#25653=CARTESIAN_POINT('Ctrl Pts',(-0.239999985886701,0.000936313964622287,
-0.00198109907211505));
#25654=CARTESIAN_POINT('Ctrl Pts',(-0.23999998754503,0.000935037276690134,
-0.00179251014885892));
#25655=CARTESIAN_POINT('Ctrl Pts',(-0.239999988374194,0.000934398932724057,
-0.00169821568723086));
#25656=CARTESIAN_POINT('Ctrl Pts',(-0.23999998888584,0.000933778680489091,
-0.001598876075407));
#25657=CARTESIAN_POINT('Ctrl Pts',(-0.239999989109537,0.000933139892818666,
-0.00148755770593738));
#25658=CARTESIAN_POINT('Ctrl Pts',(-0.239999989333234,0.000932501105148241,
-0.00137623933646776));
#25659=CARTESIAN_POINT('Ctrl Pts',(-0.23999998921348,0.000931843782075009,
-0.00125294220935238));
#25660=CARTESIAN_POINT('Ctrl Pts',(-0.239999988915679,0.000931314436538036,
-0.00114540075439106));
#25661=CARTESIAN_POINT('Ctrl Pts',(-0.239999988617877,0.000930785091001064,
-0.00103785929942974));
#25662=CARTESIAN_POINT('Ctrl Pts',(-0.239999988207469,0.000930383722896765,
-0.000946073516622472));
#25663=CARTESIAN_POINT('Ctrl Pts',(-0.239999987775988,0.000930026166834633,
-0.000851201367006931));
#25664=CARTESIAN_POINT('Ctrl Pts',(-0.239999987344506,0.000929668610772501,
-0.00075632921739139));
#25665=CARTESIAN_POINT('Ctrl Pts',(-0.239999986868716,0.000929354866792827,
-0.000658370700967577));
#25666=CARTESIAN_POINT('Ctrl Pts',(-0.239999986453847,0.000929105975935206,
-0.000562234778806111));
#25667=CARTESIAN_POINT('Ctrl Pts',(-0.239999985624108,0.000928608194219964,
-0.000369962934483178));
#25668=CARTESIAN_POINT('Ctrl Pts',(-0.239999985091289,0.000928369824712036,
-0.00018498146720963));
#25669=CARTESIAN_POINT('Ctrl Pts',(-0.239999985091289,0.000928369824712027,
4.55961963606762E-14));
#25670=CARTESIAN_POINT('Ctrl Pts',(-0.239999985091289,0.000928369824712017,
0.000184981467300823));
#25671=CARTESIAN_POINT('Ctrl Pts',(-0.239999985624108,0.000928608194219925,
0.000369962934537728));
#25672=CARTESIAN_POINT('Ctrl Pts',(-0.239999986453847,0.00092910597593532,
0.000562234778872252));
#25673=CARTESIAN_POINT('Ctrl Pts',(-0.239999986868716,0.000929354866793017,
0.000658370701039514));
#25674=CARTESIAN_POINT('Ctrl Pts',(-0.239999987344506,0.000929668610772811,
0.000756329217481181));
#25675=CARTESIAN_POINT('Ctrl Pts',(-0.239999987775988,0.000930026166834889,
0.000851201367079335));
#25676=CARTESIAN_POINT('Ctrl Pts',(-0.239999988207469,0.000930383722896967,
0.000946073516677489));
#25677=CARTESIAN_POINT('Ctrl Pts',(-0.239999988617877,0.000930785091001039,
0.00103785929943213));
#25678=CARTESIAN_POINT('Ctrl Pts',(-0.239999988915679,0.00093131443653849,
0.00114540075448225));
#25679=CARTESIAN_POINT('Ctrl Pts',(-0.23999998921348,0.000931843782075941,
0.00125294220953238));
#25680=CARTESIAN_POINT('Ctrl Pts',(-0.239999989333234,0.000932501105150358,
0.00137623933687799));
#25681=CARTESIAN_POINT('Ctrl Pts',(-0.239999989109537,0.000933139892821468,
0.0014875577064776));
#25682=CARTESIAN_POINT('Ctrl Pts',(-0.23999998888584,0.000933778680492577,
0.00159887607607722));
#25683=CARTESIAN_POINT('Ctrl Pts',(-0.239999988374194,0.000934398932727729,
0.00169821568793084));
#25684=CARTESIAN_POINT('Ctrl Pts',(-0.23999998754503,0.000935037276693792,
0.00179251014954883));
#25685=CARTESIAN_POINT('Ctrl Pts',(-0.239999985886701,0.000936313964625918,
0.00198109907278481));
#25686=CARTESIAN_POINT('Ctrl Pts',(-0.239999982890083,0.000937663019539288,
0.0021495073950783));
#25687=CARTESIAN_POINT('Ctrl Pts',(-0.239999978314326,0.000939047803401668,
0.00229080150891891));
#25688=CARTESIAN_POINT('Origin',(-0.238000089723382,0.000932439548048954,
8.085935608268E-7));
#25689=CARTESIAN_POINT('Ctrl Pts',(-0.239999996099768,0.000939047805433175,
-0.00229080150878961));
#25690=CARTESIAN_POINT('Ctrl Pts',(-0.240000043006653,0.000528617519648317,
-0.00229337348318028));
#25691=CARTESIAN_POINT('Ctrl Pts',(-0.239869494268692,0.000118749315230352,
-0.00229595732371585));
#25692=CARTESIAN_POINT('Ctrl Pts',(-0.239633235322195,-0.000215513325754126,
-0.00229850428565031));
#25693=CARTESIAN_POINT('Ctrl Pts',(-0.239569418327284,-0.000305802551093352,
-0.00229919225729845));
#25694=CARTESIAN_POINT('Ctrl Pts',(-0.239498166602568,-0.000390684708998686,
-0.0022998800374307));
#25695=CARTESIAN_POINT('Ctrl Pts',(-0.239420535407129,-0.000469012056432765,
-0.00230057142549143));
#25696=CARTESIAN_POINT('Ctrl Pts',(-0.239132270695065,-0.000759861760950644,
-0.00230313872822486));
#25697=CARTESIAN_POINT('Ctrl Pts',(-0.2387511004726,-0.000959690921395982,
-0.00230570344552429));
#25698=CARTESIAN_POINT('Ctrl Pts',(-0.238346576518808,-0.00103084593839461,
-0.00230827883574627));
#25699=CARTESIAN_POINT('Ctrl Pts',(-0.238238848668799,-0.00104979506841949,
-0.00230896468203286));
#25700=CARTESIAN_POINT('Ctrl Pts',(-0.238129594726146,-0.0010598784421159,
-0.00230965111096215));
#25701=CARTESIAN_POINT('Ctrl Pts',(-0.238020319825353,-0.00106098210578189,
-0.00231033750372615));
#25702=CARTESIAN_POINT('Ctrl Pts',(-0.238020319827727,-0.00106098234435247,
0.00231033750623555));
#25703=CARTESIAN_POINT('Ctrl Pts',(-0.238430653011175,-0.00105683802591466,
0.00230776006436476));
#25704=CARTESIAN_POINT('Ctrl Pts',(-0.238839618608655,-0.000922133765191787,
0.00230518882237866));
#25705=CARTESIAN_POINT('Ctrl Pts',(-0.239172040185025,-0.000681733222427424,
0.00230262217336099));
#25706=CARTESIAN_POINT('Ctrl Pts',(-0.239260566696896,-0.000617712644295366,
0.002301938654297));
#25707=CARTESIAN_POINT('Ctrl Pts',(-0.239343768351535,-0.00054646776209465,
0.00230125511985015));
#25708=CARTESIAN_POINT('Ctrl Pts',(-0.239420535523769,-0.000469012172569021,
0.00230057142670432));
#25709=CARTESIAN_POINT('Ctrl Pts',(-0.239707936442746,-0.000179033957119173,
0.00229801181648694));
#25710=CARTESIAN_POINT('Ctrl Pts',(-0.23990449768155,0.000202999713542514,
0.002295473453181));
#25711=CARTESIAN_POINT('Ctrl Pts',(-0.23997243007692,0.000607909087375879,
0.00229289178149579));
#25712=CARTESIAN_POINT('Ctrl Pts',(-0.239990779616387,0.000717281066604452,
0.00229219443398997));
#25713=CARTESIAN_POINT('Ctrl Pts',(-0.240000008778427,0.00082818455522576,
0.00229149623695115));
#25714=CARTESIAN_POINT('Ctrl Pts',(-0.239999996094959,0.000939047805435644,
0.00229080150888079));
#25715=CARTESIAN_POINT('Origin',(-0.237999996123667,0.00749999988066555,
0.00222451372646705));
#25716=CARTESIAN_POINT('Ctrl Pts',(-0.239999996099769,0.0140609521945749,
0.00229080150797066));
#25717=CARTESIAN_POINT('Ctrl Pts',(-0.240000043006654,0.0144713824803586,
0.00229337348232777));
#25718=CARTESIAN_POINT('Ctrl Pts',(-0.239869494268694,0.0148812506847756,
0.00229595732282965));
#25719=CARTESIAN_POINT('Ctrl Pts',(-0.239633235322198,0.0152155133257598,
0.002298504284731));
#25720=CARTESIAN_POINT('Ctrl Pts',(-0.239569418327287,0.015305802551099,
0.0022991922563702));
#25721=CARTESIAN_POINT('Ctrl Pts',(-0.239498166602572,0.0153906847090043,
0.00229988003649352));
#25722=CARTESIAN_POINT('Ctrl Pts',(-0.239420535407133,0.0154690120564384,
0.00230057142454528));
#25723=CARTESIAN_POINT('Ctrl Pts',(-0.239132270695066,0.0157598617609598,
0.00230313872724546));
#25724=CARTESIAN_POINT('Ctrl Pts',(-0.238751100472598,0.0159596909214074,
0.00230570344451184));
#25725=CARTESIAN_POINT('Ctrl Pts',(-0.238346576518801,0.0160308459384058,
0.00230827883470088));
#25726=CARTESIAN_POINT('Ctrl Pts',(-0.238238848668797,0.0160497950684295,
0.00230896468097866));
#25727=CARTESIAN_POINT('Ctrl Pts',(-0.238129594726149,0.0160598784421256,
0.00230965110989914));
#25728=CARTESIAN_POINT('Ctrl Pts',(-0.238020319825361,0.0160609821057921,
0.00231033750265435));
#25729=CARTESIAN_POINT('Origin',(-0.237999996123666,0.00750000011933441,
-0.00222451372646644));
#25730=CARTESIAN_POINT('Ctrl Pts',(-0.238020319827727,0.0160609823443528,
-0.00231033750623781));
#25731=CARTESIAN_POINT('Ctrl Pts',(-0.238430653011171,0.0160568380259149,
-0.00230776006436743));
#25732=CARTESIAN_POINT('Ctrl Pts',(-0.238839618608648,0.0159221337651943,
-0.00230518882238151));
#25733=CARTESIAN_POINT('Ctrl Pts',(-0.239172040185016,0.0156817332224338,
-0.00230262217336384));
#25734=CARTESIAN_POINT('Ctrl Pts',(-0.23926056669689,0.0156177126442999,
-0.00230193865429981));
#25735=CARTESIAN_POINT('Ctrl Pts',(-0.239343768351532,0.0155464677620968,
-0.00230125511985291));
#25736=CARTESIAN_POINT('Ctrl Pts',(-0.239420535523769,0.0154690121725683,
-0.00230057142670702));
#25737=CARTESIAN_POINT('Ctrl Pts',(-0.239707936442746,0.0151790339571179,
-0.00229801181648951));
#25738=CARTESIAN_POINT('Ctrl Pts',(-0.23990449768155,0.0147970002864556,
-0.00229547345318327));
#25739=CARTESIAN_POINT('Ctrl Pts',(-0.23997243007692,0.0143920909126221,
-0.00229289178149773));
#25740=CARTESIAN_POINT('Ctrl Pts',(-0.239990779616386,0.0142827189333941,
-0.00229219443399182));
#25741=CARTESIAN_POINT('Ctrl Pts',(-0.240000008778426,0.0141718154447735,
-0.00229149623695292));
#25742=CARTESIAN_POINT('Ctrl Pts',(-0.239999996094958,0.0140609521945643,
-0.00229080150888247));
#25743=CARTESIAN_POINT('Origin',(-0.238000089723382,0.0140675604519525,
-8.08593956556282E-7));
#25744=CARTESIAN_POINT('Origin',(-0.1795,0.0075,0.));
#25745=CARTESIAN_POINT('Origin',(-0.1795,0.0075,-0.0079756477610481));
#25746=CARTESIAN_POINT('Origin',(-0.1795,0.0075,0.));
#25747=CARTESIAN_POINT('Origin',(-0.1795,0.0075,-0.0045));
#25748=CARTESIAN_POINT('Origin',(-0.1405,0.0075,0.));
#25749=CARTESIAN_POINT('Origin',(-0.1405,0.0075,-0.0055));
#25750=CARTESIAN_POINT('Origin',(-0.1405,0.0075,0.));
#25751=CARTESIAN_POINT('Origin',(-0.1405,0.0075,-0.00882888901198444));
#25752=CARTESIAN_POINT('Origin',(-0.1406,0.0075,0.));
#25753=CARTESIAN_POINT('Origin',(-0.1406,0.0075,-0.00882888901198444));
#25754=CARTESIAN_POINT('Origin',(-0.1421,0.0075,0.));
#25755=CARTESIAN_POINT('Origin',(-0.1421,0.0075,-0.00882888901198444));
#25756=CARTESIAN_POINT('Origin',(-0.1419,0.0075,0.));
#25757=CARTESIAN_POINT('Origin',(-0.1419,0.0075,0.00882888901198444));
#25758=CARTESIAN_POINT('Origin',(-0.1436,0.0075,0.));
#25759=CARTESIAN_POINT('Origin',(-0.1436,0.0075,-0.00882888901198444));
#25760=CARTESIAN_POINT('Origin',(-0.1434,0.0075,0.));
#25761=CARTESIAN_POINT('Origin',(-0.1434,0.0075,0.00882888901198444));
#25762=CARTESIAN_POINT('Origin',(-0.1451,0.0075,0.));
#25763=CARTESIAN_POINT('Origin',(-0.1451,0.0075,-0.00882888901198444));
#25764=CARTESIAN_POINT('Origin',(-0.1449,0.0075,0.));
#25765=CARTESIAN_POINT('Origin',(-0.1449,0.0075,0.00882888901198444));
#25766=CARTESIAN_POINT('Origin',(-0.1464,0.0075,0.));
#25767=CARTESIAN_POINT('Origin',(-0.1464,0.0075,0.00882888901198444));
#25768=CARTESIAN_POINT('Origin',(-0.1466,0.0075,0.));
#25769=CARTESIAN_POINT('Origin',(-0.1466,0.0075,-0.00882888901198444));
#25770=CARTESIAN_POINT('Origin',(-0.1479,0.0075,0.));
#25771=CARTESIAN_POINT('Origin',(-0.1479,0.0075,0.00882888901198444));
#25772=CARTESIAN_POINT('Origin',(-0.149526465075064,0.0075,0.));
#25773=CARTESIAN_POINT('Origin',(-0.149526465075064,0.0075,-0.00882888901198444));
#25774=CARTESIAN_POINT('Origin',(-0.1595,0.0075,0.));
#25775=CARTESIAN_POINT('Origin',(-0.1595,0.0075,-0.00882888901198444));
#25776=CARTESIAN_POINT('Origin',(-0.159473534924936,0.0075,0.));
#25777=CARTESIAN_POINT('Origin',(-0.159473534924936,0.0075,0.00882888901198444));
#25778=CARTESIAN_POINT('Origin',(-0.158026465075064,0.0075,0.));
#25779=CARTESIAN_POINT('Origin',(-0.158026465075064,0.0075,-0.00882888901198444));
#25780=CARTESIAN_POINT('Origin',(-0.150973534924937,0.0075,0.));
#25781=CARTESIAN_POINT('Origin',(-0.150973534924937,0.0075,0.00882888901198444));
#25782=CARTESIAN_POINT('Ctrl Pts',(-0.180492715511507,0.00208357847138839,
0.00778381458262853));
#25783=CARTESIAN_POINT('Ctrl Pts',(-0.18,0.00208768551873161,0.00777792629190908));
#25784=CARTESIAN_POINT('Ctrl Pts',(-0.18,0.00236958913814357,0.00737375990977421));
#25785=CARTESIAN_POINT('Ctrl Pts',(-0.180494324020048,0.00106537901854582,
0.00707337168038232));
#25786=CARTESIAN_POINT('Ctrl Pts',(-0.18,0.00106751218715109,0.00706776299687777));
#25787=CARTESIAN_POINT('Ctrl Pts',(-0.18,0.0014052360688775,0.00670086601600097));
#25788=CARTESIAN_POINT('Ctrl Pts',(-0.180498282439035,-0.000688149212900568,
0.00524596704164286));
#25789=CARTESIAN_POINT('Ctrl Pts',(-0.18,-0.000692161918799494,0.00523579826232968));
#25790=CARTESIAN_POINT('Ctrl Pts',(-0.18,-0.000255396373108266,0.00497022946835977));
#25791=CARTESIAN_POINT('Ctrl Pts',(-0.180508571884256,-0.00206121245391611,
0.00171196042612565));
#25792=CARTESIAN_POINT('Ctrl Pts',(-0.18,-0.00207089065980965,0.0017061119940659));
#25793=CARTESIAN_POINT('Ctrl Pts',(-0.18,-0.00155636923028695,0.001622484125152));
#25794=CARTESIAN_POINT('Ctrl Pts',(-0.180507701632299,-0.00198984920249958,
-0.00207534072170255));
#25795=CARTESIAN_POINT('Ctrl Pts',(-0.18,-0.00199898872775875,-0.00206848014615668));
#25796=CARTESIAN_POINT('Ctrl Pts',(-0.18,-0.0014886043286521,-0.00196703616742313));
#25797=CARTESIAN_POINT('Ctrl Pts',(-0.180497559880866,-0.000482912630366871,
-0.00555392798696781));
#25798=CARTESIAN_POINT('Ctrl Pts',(-0.18,-0.000486526972169703,-0.00554405840433583));
#25799=CARTESIAN_POINT('Ctrl Pts',(-0.18,-6.11665353613021E-5,-0.00526163542994926));
#25800=CARTESIAN_POINT('Ctrl Pts',(-0.180491867056987,0.00224576313070539,
-0.0081898374281038));
#25801=CARTESIAN_POINT('Ctrl Pts',(-0.18,0.00224601031558402,-0.00818083867958575));
#25802=CARTESIAN_POINT('Ctrl Pts',(-0.18,0.00252313449484398,-0.00775830380791825));
#25803=CARTESIAN_POINT('Ctrl Pts',(-0.180488462887617,0.00577942932125372,
-0.00958054386633694));
#25804=CARTESIAN_POINT('Ctrl Pts',(-0.18,0.00577937831377157,-0.00956893262499887));
#25805=CARTESIAN_POINT('Ctrl Pts',(-0.18,0.00587025317906997,-0.00907572435223234));
#25806=CARTESIAN_POINT('Ctrl Pts',(-0.180488629342552,0.00957710911122243,
-0.00950944489475148));
#25807=CARTESIAN_POINT('Ctrl Pts',(-0.18,0.00957712259305036,-0.00949788380666547));
#25808=CARTESIAN_POINT('Ctrl Pts',(-0.18,0.0094675316846421,-0.00900837007444288));
#25809=CARTESIAN_POINT('Ctrl Pts',(-0.180492343722264,0.0130567083237039,
-0.00798771374964044));
#25810=CARTESIAN_POINT('Ctrl Pts',(-0.18,0.0130566470856787,-0.00797903414015096));
#25811=CARTESIAN_POINT('Ctrl Pts',(-0.18,0.0127633603172519,-0.00756679005675688));
#25812=CARTESIAN_POINT('Ctrl Pts',(-0.180498277776074,0.0156878479525759,
-0.00524728696109442));
#25813=CARTESIAN_POINT('Ctrl Pts',(-0.18,0.0156918696359066,-0.00523708434816095));
#25814=CARTESIAN_POINT('Ctrl Pts',(-0.18,0.0152551103542225,-0.00497147978047479));
#25815=CARTESIAN_POINT('Ctrl Pts',(-0.180508590057067,0.0170631420237172,
-0.00170670572622402));
#25816=CARTESIAN_POINT('Ctrl Pts',(-0.18,0.0170728417288127,-0.00170085628138549));
#25817=CARTESIAN_POINT('Ctrl Pts',(-0.18,0.0165581992152197,-0.00161750652259339));
#25818=CARTESIAN_POINT('Ctrl Pts',(-0.180507676294974,0.0169879516360366,
0.00208672420876621));
#25819=CARTESIAN_POINT('Ctrl Pts',(-0.18,0.0169970776392087,0.00207981994539201));
#25820=CARTESIAN_POINT('Ctrl Pts',(-0.18,0.0164868018720009,0.00197783354485042));
#25821=CARTESIAN_POINT('Ctrl Pts',(-0.180497532146321,0.0154750030588555,
0.00556552633006958));
#25822=CARTESIAN_POINT('Ctrl Pts',(-0.18,0.0154786081176936,0.00555565825322737));
#25823=CARTESIAN_POINT('Ctrl Pts',(-0.18,0.0150536805229185,0.00527261080601529));
#25824=CARTESIAN_POINT('Ctrl Pts',(-0.180491851706073,0.0127430969971975,
0.00819641820051746));
#25825=CARTESIAN_POINT('Ctrl Pts',(-0.18,0.0127428333825127,0.00818741797918455));
#25826=CARTESIAN_POINT('Ctrl Pts',(-0.18,0.01246631245657,0.00776454042759482));
#25827=CARTESIAN_POINT('Ctrl Pts',(-0.180488461754297,0.00921325615876769,
0.00958099954636007));
#25828=CARTESIAN_POINT('Ctrl Pts',(-0.18,0.00921330243936221,0.00956938959009847));
#25829=CARTESIAN_POINT('Ctrl Pts',(-0.18,0.00912281682762101,0.00907615564159787));
#25830=CARTESIAN_POINT('Ctrl Pts',(-0.18048863138779,0.00542104750415485,
0.00950862445512012));
#25831=CARTESIAN_POINT('Ctrl Pts',(-0.18,0.00542103959480098,0.00949706815102514));
#25832=CARTESIAN_POINT('Ctrl Pts',(-0.18,0.00553072204248816,0.00900759283099922));
#25833=CARTESIAN_POINT('Ctrl Pts',(-0.180491107002967,0.00310177792423096,
0.00849425748487474));
#25834=CARTESIAN_POINT('Ctrl Pts',(-0.18,0.00310463170987884,0.00848584310919716));
#25835=CARTESIAN_POINT('Ctrl Pts',(-0.18,0.00333394220740964,0.00804665380354745));
#25836=CARTESIAN_POINT('Ctrl Pts',(-0.180492715511507,0.00208357847138839,
0.00778381458262853));
#25837=CARTESIAN_POINT('Ctrl Pts',(-0.18,0.00208768551873161,0.00777792629190908));
#25838=CARTESIAN_POINT('Ctrl Pts',(-0.18,0.00236958913814357,0.00737375990977421));
#54551=UNCERTAINTY_MEASURE_WITH_UNIT(LENGTH_MEASURE(1.E-5),#54581,
'DISTANCE_ACCURACY_VALUE',
'Maximum model space distance between geometric entities at asserted c
onnectivities');
#54564=UNCERTAINTY_MEASURE_WITH_UNIT(LENGTH_MEASURE(1.E-5),#54581,
'DISTANCE_ACCURACY_VALUE',
'Maximum model space distance between geometric entities at asserted c
onnectivities');
#54567=(
GEOMETRIC_REPRESENTATION_CONTEXT(3)
GLOBAL_UNCERTAINTY_ASSIGNED_CONTEXT((#54551))
GLOBAL_UNIT_ASSIGNED_CONTEXT((#54581,#54582,#54583))
REPRESENTATION_CONTEXT('','3D')
);
#54580=(
GEOMETRIC_REPRESENTATION_CONTEXT(3)
GLOBAL_UNCERTAINTY_ASSIGNED_CONTEXT((#54564))
GLOBAL_UNIT_ASSIGNED_CONTEXT((#54581,#54582,#54583))
REPRESENTATION_CONTEXT('','3D')
);
#54581=(
LENGTH_UNIT()
NAMED_UNIT(*)
SI_UNIT($,.METRE.)
);
#54582=(
NAMED_UNIT(*)
PLANE_ANGLE_UNIT()
SI_UNIT($,.RADIAN.)
);
#54583=(
NAMED_UNIT(*)
SI_UNIT($,.STERADIAN.)
SOLID_ANGLE_UNIT()
);
#54586=SHAPE_DEFINITION_REPRESENTATION(#54601,#54631);
#54601=PRODUCT_DEFINITION_SHAPE('',$,#54647);
#54631=SHAPE_REPRESENTATION('',(#18394),#54567);
#54644=PRODUCT_DEFINITION_CONTEXT('part definition',#54691,'design');
#54647=PRODUCT_DEFINITION('Part_8','Part_8',#54662,#54644);
#54662=PRODUCT_DEFINITION_FORMATION('',$,#54695);
#54691=APPLICATION_CONTEXT(
'Core Data for Automotive Mechanical Design Process');
#54692=PRODUCT_CONTEXT('part definition',#54691,'mechanical');
#54695=PRODUCT('Part_8','Part_8','Part 1',(#54692));
#54710=PRESENTATION_STYLE_ASSIGNMENT((#54720));
#54711=PRESENTATION_STYLE_ASSIGNMENT((#54721));
#54712=PRESENTATION_STYLE_ASSIGNMENT((#54722));
#54720=SURFACE_STYLE_USAGE(.BOTH.,#54730);
#54721=SURFACE_STYLE_USAGE(.BOTH.,#54731);
#54722=SURFACE_STYLE_USAGE(.BOTH.,#54732);
#54730=SURFACE_SIDE_STYLE('',(#54740));
#54731=SURFACE_SIDE_STYLE('',(#54741));
#54732=SURFACE_SIDE_STYLE('',(#54742));
#54740=SURFACE_STYLE_FILL_AREA(#54750);
#54741=SURFACE_STYLE_FILL_AREA(#54751);
#54742=SURFACE_STYLE_FILL_AREA(#54752);
#54750=FILL_AREA_STYLE('Opaque(170,178,196)',(#54760));
#54751=FILL_AREA_STYLE('Opaque(229,234,237)',(#54761));
#54752=FILL_AREA_STYLE('Opaque(26,26,26)',(#54762));
#54760=FILL_AREA_STYLE_COLOUR('Opaque(170,178,196)',#54770);
#54761=FILL_AREA_STYLE_COLOUR('Opaque(229,234,237)',#54771);
#54762=FILL_AREA_STYLE_COLOUR('Opaque(26,26,26)',#54772);
#54770=COLOUR_RGB('Opaque(170,178,196)', 0.66274510, 0.83137255, 0.94901961);
#54771=COLOUR_RGB('Opaque(229,234,237)', 0.40784314, 0.44705882, 0.49803922);
#54772=COLOUR_RGB('Opaque(26,26,26)', 0.66274510, 0.83137255, 0.94901961);
ENDSEC;
END-ISO-10303-21;
